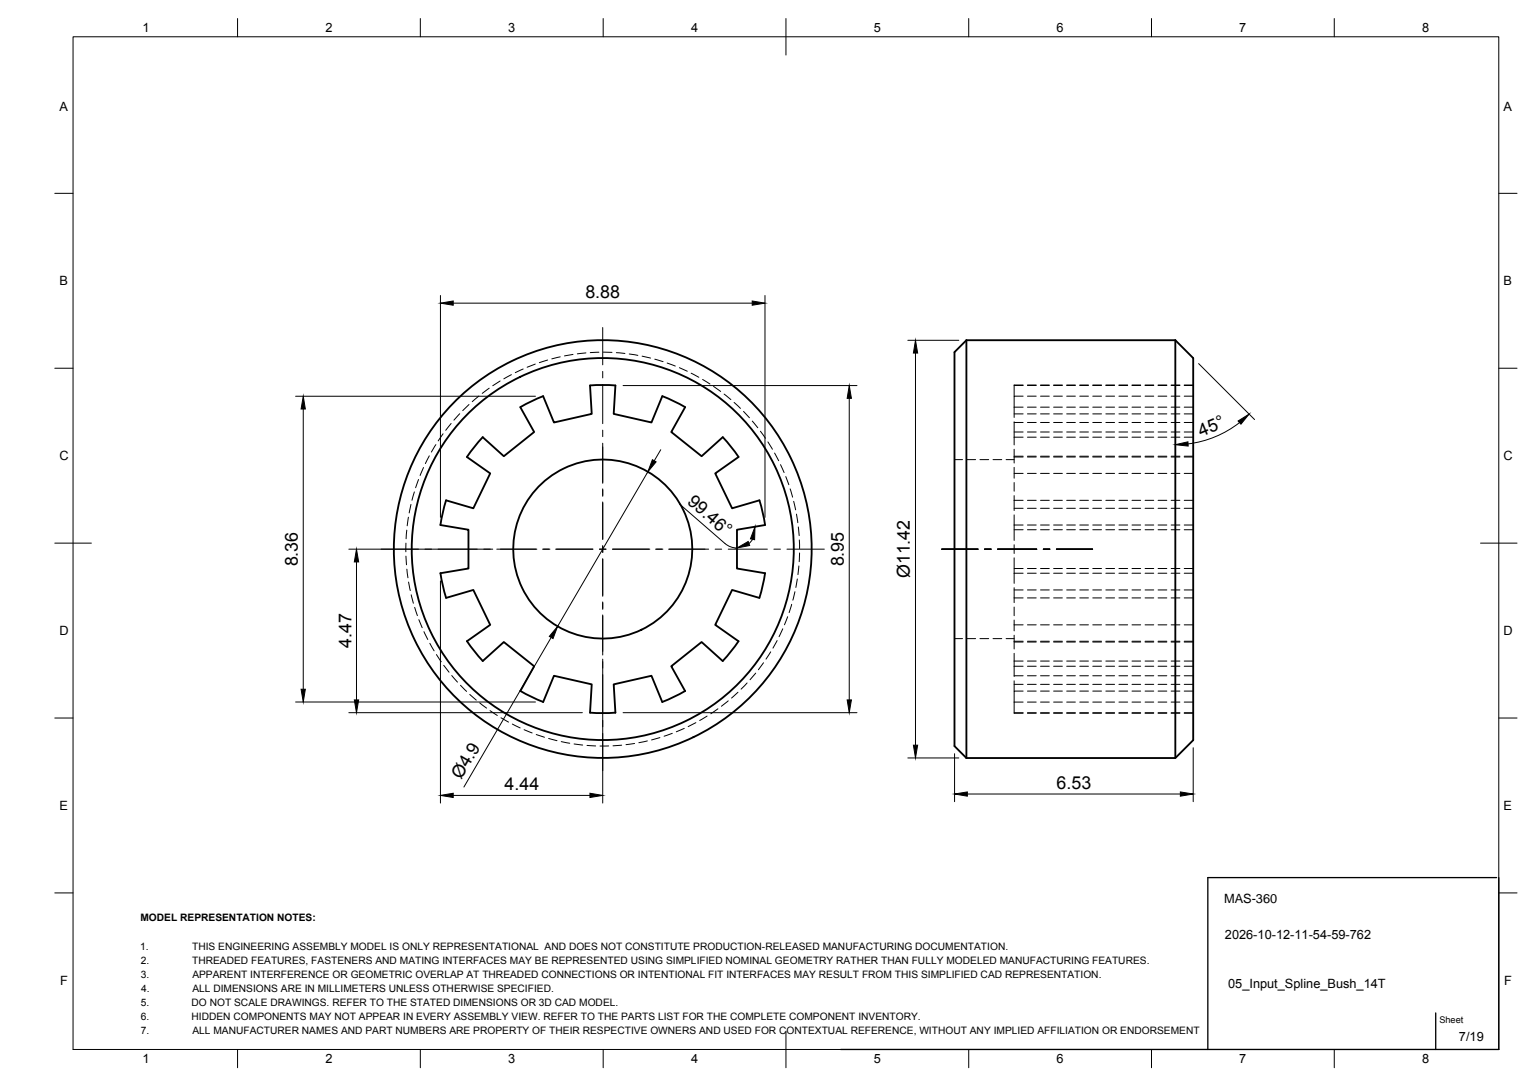
ISO-10303-21;
HEADER;
/* Generated by software containing ST-Developer
 * from STEP Tools, Inc. (www.steptools.com) 
 */

FILE_DESCRIPTION(
/* description */ (''),
/* implementation_level */ '2;1');

FILE_NAME(
/* name */ '05_Input_Spline_Bush_14T.step',
/* time_stamp */ '2026-11-04T18:53:29-08:00',
/* author */ (''),
/* organization */ (''),
/* preprocessor_version */ 'ST-DEVELOPER v20.2',
/* originating_system */ 'Autodesk Translation Framework v15.17.0.0',
/* authorisation */ '');

FILE_SCHEMA (('AUTOMOTIVE_DESIGN { 1 0 10303 214 3 1 1 }'));
ENDSEC;

DATA;
#10=MECHANICAL_DESIGN_GEOMETRIC_PRESENTATION_REPRESENTATION('',(#1331),#100031);
#230=CONICAL_SURFACE('',#21438,5.5488,0.785398163397448);
#231=CONICAL_SURFACE('',#21447,5.4672,0.785398163397448);
#748=CIRCLE('',#21439,5.712);
#749=CIRCLE('',#21440,5.3856);
#750=CIRCLE('',#21441,5.712);
#751=CIRCLE('',#21443,5.712);
#752=CIRCLE('',#21444,5.712);
#753=CIRCLE('',#21446,2.448);
#754=CIRCLE('',#21448,5.2224);
#755=CIRCLE('',#21450,4.488);
#756=CIRCLE('',#21451,4.488);
#757=CIRCLE('',#21452,4.488);
#758=CIRCLE('',#21453,4.488);
#759=CIRCLE('',#21454,4.488);
#760=CIRCLE('',#21455,4.488);
#761=CIRCLE('',#21456,4.488);
#762=CIRCLE('',#21457,4.488);
#763=CIRCLE('',#21458,4.488);
#764=CIRCLE('',#21459,4.488);
#765=CIRCLE('',#21460,4.488);
#766=CIRCLE('',#21461,4.488);
#767=CIRCLE('',#21462,4.488);
#768=CIRCLE('',#21463,4.488);
#769=CIRCLE('',#21468,4.488);
#770=CIRCLE('',#21473,4.488);
#771=CIRCLE('',#21478,4.488);
#772=CIRCLE('',#21483,4.488);
#773=CIRCLE('',#21488,4.488);
#774=CIRCLE('',#21493,4.488);
#775=CIRCLE('',#21498,4.488);
#776=CIRCLE('',#21503,4.488);
#777=CIRCLE('',#21508,4.488);
#778=CIRCLE('',#21513,4.488);
#779=CIRCLE('',#21518,4.488);
#780=CIRCLE('',#21523,4.488);
#781=CIRCLE('',#21528,4.488);
#782=CIRCLE('',#21533,4.488);
#783=CIRCLE('',#21534,2.448);
#1295=SHAPE_REPRESENTATION_RELATIONSHIP('SRR','None',#100105,#1313);
#1313=ADVANCED_BREP_SHAPE_REPRESENTATION('',(#1349),#100017);
#1331=STYLED_ITEM('',(#100200),#1349);
#1349=MANIFOLD_SOLID_BREP('Body1',#20121);
#1477=PLANE('',#21445);
#1478=PLANE('',#21449);
#1479=PLANE('',#21464);
#1480=PLANE('',#21465);
#1481=PLANE('',#21466);
#1482=PLANE('',#21469);
#1483=PLANE('',#21470);
#1484=PLANE('',#21471);
#1485=PLANE('',#21474);
#1486=PLANE('',#21475);
#1487=PLANE('',#21476);
#1488=PLANE('',#21479);
#1489=PLANE('',#21480);
#1490=PLANE('',#21481);
#1491=PLANE('',#21484);
#1492=PLANE('',#21485);
#1493=PLANE('',#21486);
#1494=PLANE('',#21489);
#1495=PLANE('',#21490);
#1496=PLANE('',#21491);
#1497=PLANE('',#21494);
#1498=PLANE('',#21495);
#1499=PLANE('',#21496);
#1500=PLANE('',#21499);
#1501=PLANE('',#21500);
#1502=PLANE('',#21501);
#1503=PLANE('',#21504);
#1504=PLANE('',#21505);
#1505=PLANE('',#21506);
#1506=PLANE('',#21509);
#1507=PLANE('',#21510);
#1508=PLANE('',#21511);
#1509=PLANE('',#21514);
#1510=PLANE('',#21515);
#1511=PLANE('',#21516);
#1512=PLANE('',#21519);
#1513=PLANE('',#21520);
#1514=PLANE('',#21521);
#1515=PLANE('',#21524);
#1516=PLANE('',#21525);
#1517=PLANE('',#21526);
#1518=PLANE('',#21529);
#1519=PLANE('',#21530);
#1520=PLANE('',#21531);
#1521=PLANE('',#21532);
#1754=FACE_BOUND('',#6840,.T.);
#1755=FACE_BOUND('',#6843,.T.);
#1756=FACE_BOUND('',#6900,.T.);
#2596=LINE('',#61632,#3883);
#2597=LINE('',#61640,#3884);
#2598=LINE('',#61646,#3885);
#2599=LINE('',#61653,#3886);
#2600=LINE('',#61655,#3887);
#2601=LINE('',#61657,#3888);
#2602=LINE('',#61661,#3889);
#2603=LINE('',#61663,#3890);
#2604=LINE('',#61665,#3891);
#2605=LINE('',#61669,#3892);
#2606=LINE('',#61671,#3893);
#2607=LINE('',#61673,#3894);
#2608=LINE('',#61677,#3895);
#2609=LINE('',#61679,#3896);
#2610=LINE('',#61681,#3897);
#2611=LINE('',#61685,#3898);
#2612=LINE('',#61687,#3899);
#2613=LINE('',#61689,#3900);
#2614=LINE('',#61693,#3901);
#2615=LINE('',#61695,#3902);
#2616=LINE('',#61697,#3903);
#2617=LINE('',#61701,#3904);
#2618=LINE('',#61703,#3905);
#2619=LINE('',#61705,#3906);
#2620=LINE('',#61709,#3907);
#2621=LINE('',#61711,#3908);
#2622=LINE('',#61713,#3909);
#2623=LINE('',#61717,#3910);
#2624=LINE('',#61719,#3911);
#2625=LINE('',#61721,#3912);
#2626=LINE('',#61725,#3913);
#2627=LINE('',#61727,#3914);
#2628=LINE('',#61729,#3915);
#2629=LINE('',#61733,#3916);
#2630=LINE('',#61735,#3917);
#2631=LINE('',#61737,#3918);
#2632=LINE('',#61741,#3919);
#2633=LINE('',#61743,#3920);
#2634=LINE('',#61745,#3921);
#2635=LINE('',#61749,#3922);
#2636=LINE('',#61751,#3923);
#2637=LINE('',#61753,#3924);
#2638=LINE('',#61757,#3925);
#2639=LINE('',#61759,#3926);
#2640=LINE('',#61760,#3927);
#2641=LINE('',#61763,#3928);
#2642=LINE('',#61765,#3929);
#2643=LINE('',#61766,#3930);
#2644=LINE('',#61769,#3931);
#2645=LINE('',#61771,#3932);
#2646=LINE('',#61772,#3933);
#2647=LINE('',#61774,#3934);
#2648=LINE('',#61778,#3935);
#2649=LINE('',#61781,#3936);
#2650=LINE('',#61782,#3937);
#2651=LINE('',#61785,#3938);
#2652=LINE('',#61787,#3939);
#2653=LINE('',#61788,#3940);
#2654=LINE('',#61790,#3941);
#2655=LINE('',#61794,#3942);
#2656=LINE('',#61797,#3943);
#2657=LINE('',#61798,#3944);
#2658=LINE('',#61801,#3945);
#2659=LINE('',#61803,#3946);
#2660=LINE('',#61804,#3947);
#2661=LINE('',#61806,#3948);
#2662=LINE('',#61810,#3949);
#2663=LINE('',#61813,#3950);
#2664=LINE('',#61814,#3951);
#2665=LINE('',#61817,#3952);
#2666=LINE('',#61819,#3953);
#2667=LINE('',#61820,#3954);
#2668=LINE('',#61822,#3955);
#2669=LINE('',#61826,#3956);
#2670=LINE('',#61829,#3957);
#2671=LINE('',#61830,#3958);
#2672=LINE('',#61833,#3959);
#2673=LINE('',#61835,#3960);
#2674=LINE('',#61836,#3961);
#2675=LINE('',#61838,#3962);
#2676=LINE('',#61842,#3963);
#2677=LINE('',#61845,#3964);
#2678=LINE('',#61846,#3965);
#2679=LINE('',#61849,#3966);
#2680=LINE('',#61851,#3967);
#2681=LINE('',#61852,#3968);
#2682=LINE('',#61854,#3969);
#2683=LINE('',#61858,#3970);
#2684=LINE('',#61861,#3971);
#2685=LINE('',#61862,#3972);
#2686=LINE('',#61865,#3973);
#2687=LINE('',#61867,#3974);
#2688=LINE('',#61868,#3975);
#2689=LINE('',#61870,#3976);
#2690=LINE('',#61874,#3977);
#2691=LINE('',#61877,#3978);
#2692=LINE('',#61878,#3979);
#2693=LINE('',#61881,#3980);
#2694=LINE('',#61883,#3981);
#2695=LINE('',#61884,#3982);
#2696=LINE('',#61886,#3983);
#2697=LINE('',#61890,#3984);
#2698=LINE('',#61893,#3985);
#2699=LINE('',#61894,#3986);
#2700=LINE('',#61897,#3987);
#2701=LINE('',#61899,#3988);
#2702=LINE('',#61900,#3989);
#2703=LINE('',#61902,#3990);
#2704=LINE('',#61906,#3991);
#2705=LINE('',#61909,#3992);
#2706=LINE('',#61910,#3993);
#2707=LINE('',#61913,#3994);
#2708=LINE('',#61915,#3995);
#2709=LINE('',#61916,#3996);
#2710=LINE('',#61918,#3997);
#2711=LINE('',#61922,#3998);
#2712=LINE('',#61925,#3999);
#2713=LINE('',#61926,#4000);
#2714=LINE('',#61929,#4001);
#2715=LINE('',#61931,#4002);
#2716=LINE('',#61932,#4003);
#2717=LINE('',#61934,#4004);
#2718=LINE('',#61938,#4005);
#2719=LINE('',#61941,#4006);
#2720=LINE('',#61942,#4007);
#2721=LINE('',#61945,#4008);
#2722=LINE('',#61947,#4009);
#2723=LINE('',#61948,#4010);
#2724=LINE('',#61950,#4011);
#2725=LINE('',#61954,#4012);
#2726=LINE('',#61957,#4013);
#2727=LINE('',#61958,#4014);
#2728=LINE('',#61961,#4015);
#2729=LINE('',#61963,#4016);
#2730=LINE('',#61964,#4017);
#2731=LINE('',#61966,#4018);
#2732=LINE('',#61970,#4019);
#2733=LINE('',#61973,#4020);
#2734=LINE('',#61975,#4021);
#2735=LINE('',#61976,#4022);
#2736=LINE('',#61979,#4023);
#2737=LINE('',#61980,#4024);
#2738=LINE('',#61982,#4025);
#2739=LINE('',#61989,#4026);
#3883=VECTOR('',#25353,5.5488);
#3884=VECTOR('',#25364,5.712);
#3885=VECTOR('',#25371,5.4672);
#3886=VECTOR('',#25378,10.);
#3887=VECTOR('',#25379,10.);
#3888=VECTOR('',#25380,10.);
#3889=VECTOR('',#25383,10.);
#3890=VECTOR('',#25384,10.);
#3891=VECTOR('',#25385,10.);
#3892=VECTOR('',#25388,10.);
#3893=VECTOR('',#25389,10.);
#3894=VECTOR('',#25390,10.);
#3895=VECTOR('',#25393,10.);
#3896=VECTOR('',#25394,10.);
#3897=VECTOR('',#25395,10.);
#3898=VECTOR('',#25398,10.);
#3899=VECTOR('',#25399,10.);
#3900=VECTOR('',#25400,10.);
#3901=VECTOR('',#25403,10.);
#3902=VECTOR('',#25404,10.);
#3903=VECTOR('',#25405,10.);
#3904=VECTOR('',#25408,10.);
#3905=VECTOR('',#25409,10.);
#3906=VECTOR('',#25410,10.);
#3907=VECTOR('',#25413,10.);
#3908=VECTOR('',#25414,10.);
#3909=VECTOR('',#25415,10.);
#3910=VECTOR('',#25418,10.);
#3911=VECTOR('',#25419,10.);
#3912=VECTOR('',#25420,10.);
#3913=VECTOR('',#25423,10.);
#3914=VECTOR('',#25424,10.);
#3915=VECTOR('',#25425,10.);
#3916=VECTOR('',#25428,10.);
#3917=VECTOR('',#25429,10.);
#3918=VECTOR('',#25430,10.);
#3919=VECTOR('',#25433,10.);
#3920=VECTOR('',#25434,10.);
#3921=VECTOR('',#25435,10.);
#3922=VECTOR('',#25438,10.);
#3923=VECTOR('',#25439,10.);
#3924=VECTOR('',#25440,10.);
#3925=VECTOR('',#25443,10.);
#3926=VECTOR('',#25444,10.);
#3927=VECTOR('',#25445,10.);
#3928=VECTOR('',#25448,10.);
#3929=VECTOR('',#25449,10.);
#3930=VECTOR('',#25450,10.);
#3931=VECTOR('',#25453,10.);
#3932=VECTOR('',#25454,10.);
#3933=VECTOR('',#25455,10.);
#3934=VECTOR('',#25458,10.);
#3935=VECTOR('',#25463,10.);
#3936=VECTOR('',#25466,10.);
#3937=VECTOR('',#25467,10.);
#3938=VECTOR('',#25470,10.);
#3939=VECTOR('',#25471,10.);
#3940=VECTOR('',#25472,10.);
#3941=VECTOR('',#25475,10.);
#3942=VECTOR('',#25480,10.);
#3943=VECTOR('',#25483,10.);
#3944=VECTOR('',#25484,10.);
#3945=VECTOR('',#25487,10.);
#3946=VECTOR('',#25488,10.);
#3947=VECTOR('',#25489,10.);
#3948=VECTOR('',#25492,10.);
#3949=VECTOR('',#25497,10.);
#3950=VECTOR('',#25500,10.);
#3951=VECTOR('',#25501,10.);
#3952=VECTOR('',#25504,10.);
#3953=VECTOR('',#25505,10.);
#3954=VECTOR('',#25506,10.);
#3955=VECTOR('',#25509,10.);
#3956=VECTOR('',#25514,10.);
#3957=VECTOR('',#25517,10.);
#3958=VECTOR('',#25518,10.);
#3959=VECTOR('',#25521,10.);
#3960=VECTOR('',#25522,10.);
#3961=VECTOR('',#25523,10.);
#3962=VECTOR('',#25526,10.);
#3963=VECTOR('',#25531,10.);
#3964=VECTOR('',#25534,10.);
#3965=VECTOR('',#25535,10.);
#3966=VECTOR('',#25538,10.);
#3967=VECTOR('',#25539,10.);
#3968=VECTOR('',#25540,10.);
#3969=VECTOR('',#25543,10.);
#3970=VECTOR('',#25548,10.);
#3971=VECTOR('',#25551,10.);
#3972=VECTOR('',#25552,10.);
#3973=VECTOR('',#25555,10.);
#3974=VECTOR('',#25556,10.);
#3975=VECTOR('',#25557,10.);
#3976=VECTOR('',#25560,10.);
#3977=VECTOR('',#25565,10.);
#3978=VECTOR('',#25568,10.);
#3979=VECTOR('',#25569,10.);
#3980=VECTOR('',#25572,10.);
#3981=VECTOR('',#25573,10.);
#3982=VECTOR('',#25574,10.);
#3983=VECTOR('',#25577,10.);
#3984=VECTOR('',#25582,10.);
#3985=VECTOR('',#25585,10.);
#3986=VECTOR('',#25586,10.);
#3987=VECTOR('',#25589,10.);
#3988=VECTOR('',#25590,10.);
#3989=VECTOR('',#25591,10.);
#3990=VECTOR('',#25594,10.);
#3991=VECTOR('',#25599,10.);
#3992=VECTOR('',#25602,10.);
#3993=VECTOR('',#25603,10.);
#3994=VECTOR('',#25606,10.);
#3995=VECTOR('',#25607,10.);
#3996=VECTOR('',#25608,10.);
#3997=VECTOR('',#25611,10.);
#3998=VECTOR('',#25616,10.);
#3999=VECTOR('',#25619,10.);
#4000=VECTOR('',#25620,10.);
#4001=VECTOR('',#25623,10.);
#4002=VECTOR('',#25624,10.);
#4003=VECTOR('',#25625,10.);
#4004=VECTOR('',#25628,10.);
#4005=VECTOR('',#25633,10.);
#4006=VECTOR('',#25636,10.);
#4007=VECTOR('',#25637,10.);
#4008=VECTOR('',#25640,10.);
#4009=VECTOR('',#25641,10.);
#4010=VECTOR('',#25642,10.);
#4011=VECTOR('',#25645,10.);
#4012=VECTOR('',#25650,10.);
#4013=VECTOR('',#25653,10.);
#4014=VECTOR('',#25654,10.);
#4015=VECTOR('',#25657,10.);
#4016=VECTOR('',#25658,10.);
#4017=VECTOR('',#25659,10.);
#4018=VECTOR('',#25662,10.);
#4019=VECTOR('',#25667,10.);
#4020=VECTOR('',#25670,10.);
#4021=VECTOR('',#25671,10.);
#4022=VECTOR('',#25672,10.);
#4023=VECTOR('',#25675,10.);
#4024=VECTOR('',#25676,10.);
#4025=VECTOR('',#25679,10.);
#4026=VECTOR('',#25690,2.448);
#4801=CYLINDRICAL_SURFACE('',#21442,5.712);
#4802=CYLINDRICAL_SURFACE('',#21467,4.488);
#4803=CYLINDRICAL_SURFACE('',#21472,4.488);
#4804=CYLINDRICAL_SURFACE('',#21477,4.488);
#4805=CYLINDRICAL_SURFACE('',#21482,4.488);
#4806=CYLINDRICAL_SURFACE('',#21487,4.488);
#4807=CYLINDRICAL_SURFACE('',#21492,4.488);
#4808=CYLINDRICAL_SURFACE('',#21497,4.488);
#4809=CYLINDRICAL_SURFACE('',#21502,4.488);
#4810=CYLINDRICAL_SURFACE('',#21507,4.488);
#4811=CYLINDRICAL_SURFACE('',#21512,4.488);
#4812=CYLINDRICAL_SURFACE('',#21517,4.488);
#4813=CYLINDRICAL_SURFACE('',#21522,4.488);
#4814=CYLINDRICAL_SURFACE('',#21527,4.488);
#4815=CYLINDRICAL_SURFACE('',#21535,4.488);
#4816=CYLINDRICAL_SURFACE('',#21536,2.448);
#5620=FACE_OUTER_BOUND('',#6837,.T.);
#5621=FACE_OUTER_BOUND('',#6838,.T.);
#5622=FACE_OUTER_BOUND('',#6839,.T.);
#5623=FACE_OUTER_BOUND('',#6841,.T.);
#5624=FACE_OUTER_BOUND('',#6842,.T.);
#5625=FACE_OUTER_BOUND('',#6844,.T.);
#5626=FACE_OUTER_BOUND('',#6845,.T.);
#5627=FACE_OUTER_BOUND('',#6846,.T.);
#5628=FACE_OUTER_BOUND('',#6847,.T.);
#5629=FACE_OUTER_BOUND('',#6848,.T.);
#5630=FACE_OUTER_BOUND('',#6849,.T.);
#5631=FACE_OUTER_BOUND('',#6850,.T.);
#5632=FACE_OUTER_BOUND('',#6851,.T.);
#5633=FACE_OUTER_BOUND('',#6852,.T.);
#5634=FACE_OUTER_BOUND('',#6853,.T.);
#5635=FACE_OUTER_BOUND('',#6854,.T.);
#5636=FACE_OUTER_BOUND('',#6855,.T.);
#5637=FACE_OUTER_BOUND('',#6856,.T.);
#5638=FACE_OUTER_BOUND('',#6857,.T.);
#5639=FACE_OUTER_BOUND('',#6858,.T.);
#5640=FACE_OUTER_BOUND('',#6859,.T.);
#5641=FACE_OUTER_BOUND('',#6860,.T.);
#5642=FACE_OUTER_BOUND('',#6861,.T.);
#5643=FACE_OUTER_BOUND('',#6862,.T.);
#5644=FACE_OUTER_BOUND('',#6863,.T.);
#5645=FACE_OUTER_BOUND('',#6864,.T.);
#5646=FACE_OUTER_BOUND('',#6865,.T.);
#5647=FACE_OUTER_BOUND('',#6866,.T.);
#5648=FACE_OUTER_BOUND('',#6867,.T.);
#5649=FACE_OUTER_BOUND('',#6868,.T.);
#5650=FACE_OUTER_BOUND('',#6869,.T.);
#5651=FACE_OUTER_BOUND('',#6870,.T.);
#5652=FACE_OUTER_BOUND('',#6871,.T.);
#5653=FACE_OUTER_BOUND('',#6872,.T.);
#5654=FACE_OUTER_BOUND('',#6873,.T.);
#5655=FACE_OUTER_BOUND('',#6874,.T.);
#5656=FACE_OUTER_BOUND('',#6875,.T.);
#5657=FACE_OUTER_BOUND('',#6876,.T.);
#5658=FACE_OUTER_BOUND('',#6877,.T.);
#5659=FACE_OUTER_BOUND('',#6878,.T.);
#5660=FACE_OUTER_BOUND('',#6879,.T.);
#5661=FACE_OUTER_BOUND('',#6880,.T.);
#5662=FACE_OUTER_BOUND('',#6881,.T.);
#5663=FACE_OUTER_BOUND('',#6882,.T.);
#5664=FACE_OUTER_BOUND('',#6883,.T.);
#5665=FACE_OUTER_BOUND('',#6884,.T.);
#5666=FACE_OUTER_BOUND('',#6885,.T.);
#5667=FACE_OUTER_BOUND('',#6886,.T.);
#5668=FACE_OUTER_BOUND('',#6887,.T.);
#5669=FACE_OUTER_BOUND('',#6888,.T.);
#5670=FACE_OUTER_BOUND('',#6889,.T.);
#5671=FACE_OUTER_BOUND('',#6890,.T.);
#5672=FACE_OUTER_BOUND('',#6891,.T.);
#5673=FACE_OUTER_BOUND('',#6892,.T.);
#5674=FACE_OUTER_BOUND('',#6893,.T.);
#5675=FACE_OUTER_BOUND('',#6894,.T.);
#5676=FACE_OUTER_BOUND('',#6895,.T.);
#5677=FACE_OUTER_BOUND('',#6896,.T.);
#5678=FACE_OUTER_BOUND('',#6897,.T.);
#5679=FACE_OUTER_BOUND('',#6898,.T.);
#5680=FACE_OUTER_BOUND('',#6899,.T.);
#5681=FACE_OUTER_BOUND('',#6901,.T.);
#5682=FACE_OUTER_BOUND('',#6902,.T.);
#6837=EDGE_LOOP('',(#15791,#15792,#15793,#15794,#15795));
#6838=EDGE_LOOP('',(#15796,#15797,#15798,#15799,#15800,#15801));
#6839=EDGE_LOOP('',(#15802));
#6840=EDGE_LOOP('',(#15803));
#6841=EDGE_LOOP('',(#15804,#15805,#15806,#15807,#15808));
#6842=EDGE_LOOP('',(#15809));
#6843=EDGE_LOOP('',(#15810,#15811,#15812,#15813,#15814,#15815,#15816,#15817,
#15818,#15819,#15820,#15821,#15822,#15823,#15824,#15825,#15826,#15827,#15828,
#15829,#15830,#15831,#15832,#15833,#15834,#15835,#15836,#15837,#15838,#15839,
#15840,#15841,#15842,#15843,#15844,#15845,#15846,#15847,#15848,#15849,#15850,
#15851,#15852,#15853,#15854,#15855,#15856,#15857,#15858,#15859,#15860,#15861,
#15862,#15863,#15864,#15865));
#6844=EDGE_LOOP('',(#15866,#15867,#15868,#15869));
#6845=EDGE_LOOP('',(#15870,#15871,#15872,#15873));
#6846=EDGE_LOOP('',(#15874,#15875,#15876,#15877));
#6847=EDGE_LOOP('',(#15878,#15879,#15880,#15881));
#6848=EDGE_LOOP('',(#15882,#15883,#15884,#15885));
#6849=EDGE_LOOP('',(#15886,#15887,#15888,#15889));
#6850=EDGE_LOOP('',(#15890,#15891,#15892,#15893));
#6851=EDGE_LOOP('',(#15894,#15895,#15896,#15897));
#6852=EDGE_LOOP('',(#15898,#15899,#15900,#15901));
#6853=EDGE_LOOP('',(#15902,#15903,#15904,#15905));
#6854=EDGE_LOOP('',(#15906,#15907,#15908,#15909));
#6855=EDGE_LOOP('',(#15910,#15911,#15912,#15913));
#6856=EDGE_LOOP('',(#15914,#15915,#15916,#15917));
#6857=EDGE_LOOP('',(#15918,#15919,#15920,#15921));
#6858=EDGE_LOOP('',(#15922,#15923,#15924,#15925));
#6859=EDGE_LOOP('',(#15926,#15927,#15928,#15929));
#6860=EDGE_LOOP('',(#15930,#15931,#15932,#15933));
#6861=EDGE_LOOP('',(#15934,#15935,#15936,#15937));
#6862=EDGE_LOOP('',(#15938,#15939,#15940,#15941));
#6863=EDGE_LOOP('',(#15942,#15943,#15944,#15945));
#6864=EDGE_LOOP('',(#15946,#15947,#15948,#15949));
#6865=EDGE_LOOP('',(#15950,#15951,#15952,#15953));
#6866=EDGE_LOOP('',(#15954,#15955,#15956,#15957));
#6867=EDGE_LOOP('',(#15958,#15959,#15960,#15961));
#6868=EDGE_LOOP('',(#15962,#15963,#15964,#15965));
#6869=EDGE_LOOP('',(#15966,#15967,#15968,#15969));
#6870=EDGE_LOOP('',(#15970,#15971,#15972,#15973));
#6871=EDGE_LOOP('',(#15974,#15975,#15976,#15977));
#6872=EDGE_LOOP('',(#15978,#15979,#15980,#15981));
#6873=EDGE_LOOP('',(#15982,#15983,#15984,#15985));
#6874=EDGE_LOOP('',(#15986,#15987,#15988,#15989));
#6875=EDGE_LOOP('',(#15990,#15991,#15992,#15993));
#6876=EDGE_LOOP('',(#15994,#15995,#15996,#15997));
#6877=EDGE_LOOP('',(#15998,#15999,#16000,#16001));
#6878=EDGE_LOOP('',(#16002,#16003,#16004,#16005));
#6879=EDGE_LOOP('',(#16006,#16007,#16008,#16009));
#6880=EDGE_LOOP('',(#16010,#16011,#16012,#16013));
#6881=EDGE_LOOP('',(#16014,#16015,#16016,#16017));
#6882=EDGE_LOOP('',(#16018,#16019,#16020,#16021));
#6883=EDGE_LOOP('',(#16022,#16023,#16024,#16025));
#6884=EDGE_LOOP('',(#16026,#16027,#16028,#16029));
#6885=EDGE_LOOP('',(#16030,#16031,#16032,#16033));
#6886=EDGE_LOOP('',(#16034,#16035,#16036,#16037));
#6887=EDGE_LOOP('',(#16038,#16039,#16040,#16041));
#6888=EDGE_LOOP('',(#16042,#16043,#16044,#16045));
#6889=EDGE_LOOP('',(#16046,#16047,#16048,#16049));
#6890=EDGE_LOOP('',(#16050,#16051,#16052,#16053));
#6891=EDGE_LOOP('',(#16054,#16055,#16056,#16057));
#6892=EDGE_LOOP('',(#16058,#16059,#16060,#16061));
#6893=EDGE_LOOP('',(#16062,#16063,#16064,#16065));
#6894=EDGE_LOOP('',(#16066,#16067,#16068,#16069));
#6895=EDGE_LOOP('',(#16070,#16071,#16072,#16073));
#6896=EDGE_LOOP('',(#16074,#16075,#16076,#16077));
#6897=EDGE_LOOP('',(#16078,#16079,#16080,#16081));
#6898=EDGE_LOOP('',(#16082,#16083,#16084,#16085));
#6899=EDGE_LOOP('',(#16086,#16087,#16088,#16089,#16090,#16091,#16092,#16093,
#16094,#16095,#16096,#16097,#16098,#16099,#16100,#16101,#16102,#16103,#16104,
#16105,#16106,#16107,#16108,#16109,#16110,#16111,#16112,#16113,#16114,#16115,
#16116,#16117,#16118,#16119,#16120,#16121,#16122,#16123,#16124,#16125,#16126,
#16127,#16128,#16129,#16130,#16131,#16132,#16133,#16134,#16135,#16136,#16137,
#16138,#16139,#16140,#16141));
#6900=EDGE_LOOP('',(#16142));
#6901=EDGE_LOOP('',(#16143,#16144,#16145,#16146));
#6902=EDGE_LOOP('',(#16147,#16148,#16149,#16150));
#8915=VERTEX_POINT('',#61628);
#8916=VERTEX_POINT('',#61629);
#8917=VERTEX_POINT('',#61631);
#8918=VERTEX_POINT('',#61636);
#8919=VERTEX_POINT('',#61637);
#8920=VERTEX_POINT('',#61642);
#8921=VERTEX_POINT('',#61645);
#8922=VERTEX_POINT('',#61649);
#8923=VERTEX_POINT('',#61650);
#8924=VERTEX_POINT('',#61652);
#8925=VERTEX_POINT('',#61654);
#8926=VERTEX_POINT('',#61656);
#8927=VERTEX_POINT('',#61658);
#8928=VERTEX_POINT('',#61660);
#8929=VERTEX_POINT('',#61662);
#8930=VERTEX_POINT('',#61664);
#8931=VERTEX_POINT('',#61666);
#8932=VERTEX_POINT('',#61668);
#8933=VERTEX_POINT('',#61670);
#8934=VERTEX_POINT('',#61672);
#8935=VERTEX_POINT('',#61674);
#8936=VERTEX_POINT('',#61676);
#8937=VERTEX_POINT('',#61678);
#8938=VERTEX_POINT('',#61680);
#8939=VERTEX_POINT('',#61682);
#8940=VERTEX_POINT('',#61684);
#8941=VERTEX_POINT('',#61686);
#8942=VERTEX_POINT('',#61688);
#8943=VERTEX_POINT('',#61690);
#8944=VERTEX_POINT('',#61692);
#8945=VERTEX_POINT('',#61694);
#8946=VERTEX_POINT('',#61696);
#8947=VERTEX_POINT('',#61698);
#8948=VERTEX_POINT('',#61700);
#8949=VERTEX_POINT('',#61702);
#8950=VERTEX_POINT('',#61704);
#8951=VERTEX_POINT('',#61706);
#8952=VERTEX_POINT('',#61708);
#8953=VERTEX_POINT('',#61710);
#8954=VERTEX_POINT('',#61712);
#8955=VERTEX_POINT('',#61714);
#8956=VERTEX_POINT('',#61716);
#8957=VERTEX_POINT('',#61718);
#8958=VERTEX_POINT('',#61720);
#8959=VERTEX_POINT('',#61722);
#8960=VERTEX_POINT('',#61724);
#8961=VERTEX_POINT('',#61726);
#8962=VERTEX_POINT('',#61728);
#8963=VERTEX_POINT('',#61730);
#8964=VERTEX_POINT('',#61732);
#8965=VERTEX_POINT('',#61734);
#8966=VERTEX_POINT('',#61736);
#8967=VERTEX_POINT('',#61738);
#8968=VERTEX_POINT('',#61740);
#8969=VERTEX_POINT('',#61742);
#8970=VERTEX_POINT('',#61744);
#8971=VERTEX_POINT('',#61746);
#8972=VERTEX_POINT('',#61748);
#8973=VERTEX_POINT('',#61750);
#8974=VERTEX_POINT('',#61752);
#8975=VERTEX_POINT('',#61754);
#8976=VERTEX_POINT('',#61756);
#8977=VERTEX_POINT('',#61758);
#8978=VERTEX_POINT('',#61762);
#8979=VERTEX_POINT('',#61764);
#8980=VERTEX_POINT('',#61768);
#8981=VERTEX_POINT('',#61770);
#8982=VERTEX_POINT('',#61776);
#8983=VERTEX_POINT('',#61780);
#8984=VERTEX_POINT('',#61784);
#8985=VERTEX_POINT('',#61786);
#8986=VERTEX_POINT('',#61792);
#8987=VERTEX_POINT('',#61796);
#8988=VERTEX_POINT('',#61800);
#8989=VERTEX_POINT('',#61802);
#8990=VERTEX_POINT('',#61808);
#8991=VERTEX_POINT('',#61812);
#8992=VERTEX_POINT('',#61816);
#8993=VERTEX_POINT('',#61818);
#8994=VERTEX_POINT('',#61824);
#8995=VERTEX_POINT('',#61828);
#8996=VERTEX_POINT('',#61832);
#8997=VERTEX_POINT('',#61834);
#8998=VERTEX_POINT('',#61840);
#8999=VERTEX_POINT('',#61844);
#9000=VERTEX_POINT('',#61848);
#9001=VERTEX_POINT('',#61850);
#9002=VERTEX_POINT('',#61856);
#9003=VERTEX_POINT('',#61860);
#9004=VERTEX_POINT('',#61864);
#9005=VERTEX_POINT('',#61866);
#9006=VERTEX_POINT('',#61872);
#9007=VERTEX_POINT('',#61876);
#9008=VERTEX_POINT('',#61880);
#9009=VERTEX_POINT('',#61882);
#9010=VERTEX_POINT('',#61888);
#9011=VERTEX_POINT('',#61892);
#9012=VERTEX_POINT('',#61896);
#9013=VERTEX_POINT('',#61898);
#9014=VERTEX_POINT('',#61904);
#9015=VERTEX_POINT('',#61908);
#9016=VERTEX_POINT('',#61912);
#9017=VERTEX_POINT('',#61914);
#9018=VERTEX_POINT('',#61920);
#9019=VERTEX_POINT('',#61924);
#9020=VERTEX_POINT('',#61928);
#9021=VERTEX_POINT('',#61930);
#9022=VERTEX_POINT('',#61936);
#9023=VERTEX_POINT('',#61940);
#9024=VERTEX_POINT('',#61944);
#9025=VERTEX_POINT('',#61946);
#9026=VERTEX_POINT('',#61952);
#9027=VERTEX_POINT('',#61956);
#9028=VERTEX_POINT('',#61960);
#9029=VERTEX_POINT('',#61962);
#9030=VERTEX_POINT('',#61968);
#9031=VERTEX_POINT('',#61972);
#9032=VERTEX_POINT('',#61974);
#9033=VERTEX_POINT('',#61978);
#9034=VERTEX_POINT('',#61985);
#11370=EDGE_CURVE('',#8915,#8916,#748,.T.);
#11371=EDGE_CURVE('',#8916,#8917,#2596,.T.);
#11372=EDGE_CURVE('',#8917,#8917,#749,.T.);
#11373=EDGE_CURVE('',#8916,#8915,#750,.T.);
#11374=EDGE_CURVE('',#8918,#8919,#751,.T.);
#11375=EDGE_CURVE('',#8919,#8918,#752,.T.);
#11376=EDGE_CURVE('',#8919,#8915,#2597,.T.);
#11377=EDGE_CURVE('',#8920,#8920,#753,.T.);
#11378=EDGE_CURVE('',#8918,#8921,#2598,.T.);
#11379=EDGE_CURVE('',#8921,#8921,#754,.T.);
#11380=EDGE_CURVE('',#8922,#8923,#755,.T.);
#11381=EDGE_CURVE('',#8923,#8924,#2599,.T.);
#11382=EDGE_CURVE('',#8924,#8925,#2600,.T.);
#11383=EDGE_CURVE('',#8925,#8926,#2601,.T.);
#11384=EDGE_CURVE('',#8926,#8927,#756,.T.);
#11385=EDGE_CURVE('',#8927,#8928,#2602,.T.);
#11386=EDGE_CURVE('',#8928,#8929,#2603,.T.);
#11387=EDGE_CURVE('',#8929,#8930,#2604,.T.);
#11388=EDGE_CURVE('',#8930,#8931,#757,.T.);
#11389=EDGE_CURVE('',#8931,#8932,#2605,.T.);
#11390=EDGE_CURVE('',#8932,#8933,#2606,.T.);
#11391=EDGE_CURVE('',#8933,#8934,#2607,.T.);
#11392=EDGE_CURVE('',#8934,#8935,#758,.T.);
#11393=EDGE_CURVE('',#8935,#8936,#2608,.T.);
#11394=EDGE_CURVE('',#8936,#8937,#2609,.T.);
#11395=EDGE_CURVE('',#8937,#8938,#2610,.T.);
#11396=EDGE_CURVE('',#8938,#8939,#759,.T.);
#11397=EDGE_CURVE('',#8939,#8940,#2611,.T.);
#11398=EDGE_CURVE('',#8940,#8941,#2612,.T.);
#11399=EDGE_CURVE('',#8941,#8942,#2613,.T.);
#11400=EDGE_CURVE('',#8942,#8943,#760,.T.);
#11401=EDGE_CURVE('',#8943,#8944,#2614,.T.);
#11402=EDGE_CURVE('',#8944,#8945,#2615,.T.);
#11403=EDGE_CURVE('',#8945,#8946,#2616,.T.);
#11404=EDGE_CURVE('',#8946,#8947,#761,.T.);
#11405=EDGE_CURVE('',#8947,#8948,#2617,.T.);
#11406=EDGE_CURVE('',#8948,#8949,#2618,.T.);
#11407=EDGE_CURVE('',#8949,#8950,#2619,.T.);
#11408=EDGE_CURVE('',#8950,#8951,#762,.T.);
#11409=EDGE_CURVE('',#8951,#8952,#2620,.T.);
#11410=EDGE_CURVE('',#8952,#8953,#2621,.T.);
#11411=EDGE_CURVE('',#8953,#8954,#2622,.T.);
#11412=EDGE_CURVE('',#8954,#8955,#763,.T.);
#11413=EDGE_CURVE('',#8955,#8956,#2623,.T.);
#11414=EDGE_CURVE('',#8956,#8957,#2624,.T.);
#11415=EDGE_CURVE('',#8957,#8958,#2625,.T.);
#11416=EDGE_CURVE('',#8958,#8959,#764,.T.);
#11417=EDGE_CURVE('',#8959,#8960,#2626,.T.);
#11418=EDGE_CURVE('',#8960,#8961,#2627,.T.);
#11419=EDGE_CURVE('',#8961,#8962,#2628,.T.);
#11420=EDGE_CURVE('',#8962,#8963,#765,.T.);
#11421=EDGE_CURVE('',#8963,#8964,#2629,.T.);
#11422=EDGE_CURVE('',#8964,#8965,#2630,.T.);
#11423=EDGE_CURVE('',#8965,#8966,#2631,.T.);
#11424=EDGE_CURVE('',#8966,#8967,#766,.T.);
#11425=EDGE_CURVE('',#8967,#8968,#2632,.T.);
#11426=EDGE_CURVE('',#8968,#8969,#2633,.T.);
#11427=EDGE_CURVE('',#8969,#8970,#2634,.T.);
#11428=EDGE_CURVE('',#8970,#8971,#767,.T.);
#11429=EDGE_CURVE('',#8971,#8972,#2635,.T.);
#11430=EDGE_CURVE('',#8972,#8973,#2636,.T.);
#11431=EDGE_CURVE('',#8973,#8974,#2637,.T.);
#11432=EDGE_CURVE('',#8974,#8975,#768,.T.);
#11433=EDGE_CURVE('',#8975,#8976,#2638,.T.);
#11434=EDGE_CURVE('',#8976,#8977,#2639,.T.);
#11435=EDGE_CURVE('',#8977,#8922,#2640,.T.);
#11436=EDGE_CURVE('',#8978,#8975,#2641,.T.);
#11437=EDGE_CURVE('',#8979,#8978,#2642,.T.);
#11438=EDGE_CURVE('',#8979,#8976,#2643,.T.);
#11439=EDGE_CURVE('',#8922,#8980,#2644,.T.);
#11440=EDGE_CURVE('',#8981,#8977,#2645,.T.);
#11441=EDGE_CURVE('',#8980,#8981,#2646,.T.);
#11442=EDGE_CURVE('',#8981,#8979,#2647,.T.);
#11443=EDGE_CURVE('',#8982,#8980,#769,.T.);
#11444=EDGE_CURVE('',#8982,#8923,#2648,.T.);
#11445=EDGE_CURVE('',#8983,#8982,#2649,.T.);
#11446=EDGE_CURVE('',#8983,#8924,#2650,.T.);
#11447=EDGE_CURVE('',#8926,#8984,#2651,.T.);
#11448=EDGE_CURVE('',#8985,#8925,#2652,.T.);
#11449=EDGE_CURVE('',#8984,#8985,#2653,.T.);
#11450=EDGE_CURVE('',#8985,#8983,#2654,.T.);
#11451=EDGE_CURVE('',#8986,#8984,#770,.T.);
#11452=EDGE_CURVE('',#8986,#8927,#2655,.T.);
#11453=EDGE_CURVE('',#8987,#8986,#2656,.T.);
#11454=EDGE_CURVE('',#8987,#8928,#2657,.T.);
#11455=EDGE_CURVE('',#8930,#8988,#2658,.T.);
#11456=EDGE_CURVE('',#8989,#8929,#2659,.T.);
#11457=EDGE_CURVE('',#8988,#8989,#2660,.T.);
#11458=EDGE_CURVE('',#8989,#8987,#2661,.T.);
#11459=EDGE_CURVE('',#8990,#8988,#771,.T.);
#11460=EDGE_CURVE('',#8990,#8931,#2662,.T.);
#11461=EDGE_CURVE('',#8991,#8990,#2663,.T.);
#11462=EDGE_CURVE('',#8991,#8932,#2664,.T.);
#11463=EDGE_CURVE('',#8934,#8992,#2665,.T.);
#11464=EDGE_CURVE('',#8993,#8933,#2666,.T.);
#11465=EDGE_CURVE('',#8992,#8993,#2667,.T.);
#11466=EDGE_CURVE('',#8993,#8991,#2668,.T.);
#11467=EDGE_CURVE('',#8994,#8992,#772,.T.);
#11468=EDGE_CURVE('',#8994,#8935,#2669,.T.);
#11469=EDGE_CURVE('',#8995,#8994,#2670,.T.);
#11470=EDGE_CURVE('',#8995,#8936,#2671,.T.);
#11471=EDGE_CURVE('',#8938,#8996,#2672,.T.);
#11472=EDGE_CURVE('',#8997,#8937,#2673,.T.);
#11473=EDGE_CURVE('',#8996,#8997,#2674,.T.);
#11474=EDGE_CURVE('',#8997,#8995,#2675,.T.);
#11475=EDGE_CURVE('',#8998,#8996,#773,.T.);
#11476=EDGE_CURVE('',#8998,#8939,#2676,.T.);
#11477=EDGE_CURVE('',#8999,#8998,#2677,.T.);
#11478=EDGE_CURVE('',#8999,#8940,#2678,.T.);
#11479=EDGE_CURVE('',#8942,#9000,#2679,.T.);
#11480=EDGE_CURVE('',#9001,#8941,#2680,.T.);
#11481=EDGE_CURVE('',#9000,#9001,#2681,.T.);
#11482=EDGE_CURVE('',#9001,#8999,#2682,.T.);
#11483=EDGE_CURVE('',#9002,#9000,#774,.T.);
#11484=EDGE_CURVE('',#9002,#8943,#2683,.T.);
#11485=EDGE_CURVE('',#9003,#9002,#2684,.T.);
#11486=EDGE_CURVE('',#9003,#8944,#2685,.T.);
#11487=EDGE_CURVE('',#8946,#9004,#2686,.T.);
#11488=EDGE_CURVE('',#9005,#8945,#2687,.T.);
#11489=EDGE_CURVE('',#9004,#9005,#2688,.T.);
#11490=EDGE_CURVE('',#9005,#9003,#2689,.T.);
#11491=EDGE_CURVE('',#9006,#9004,#775,.T.);
#11492=EDGE_CURVE('',#9006,#8947,#2690,.T.);
#11493=EDGE_CURVE('',#9007,#9006,#2691,.T.);
#11494=EDGE_CURVE('',#9007,#8948,#2692,.T.);
#11495=EDGE_CURVE('',#8950,#9008,#2693,.T.);
#11496=EDGE_CURVE('',#9009,#8949,#2694,.T.);
#11497=EDGE_CURVE('',#9008,#9009,#2695,.T.);
#11498=EDGE_CURVE('',#9009,#9007,#2696,.T.);
#11499=EDGE_CURVE('',#9010,#9008,#776,.T.);
#11500=EDGE_CURVE('',#9010,#8951,#2697,.T.);
#11501=EDGE_CURVE('',#9011,#9010,#2698,.T.);
#11502=EDGE_CURVE('',#9011,#8952,#2699,.T.);
#11503=EDGE_CURVE('',#8954,#9012,#2700,.T.);
#11504=EDGE_CURVE('',#9013,#8953,#2701,.T.);
#11505=EDGE_CURVE('',#9012,#9013,#2702,.T.);
#11506=EDGE_CURVE('',#9013,#9011,#2703,.T.);
#11507=EDGE_CURVE('',#9014,#9012,#777,.T.);
#11508=EDGE_CURVE('',#9014,#8955,#2704,.T.);
#11509=EDGE_CURVE('',#9015,#9014,#2705,.T.);
#11510=EDGE_CURVE('',#9015,#8956,#2706,.T.);
#11511=EDGE_CURVE('',#8958,#9016,#2707,.T.);
#11512=EDGE_CURVE('',#9017,#8957,#2708,.T.);
#11513=EDGE_CURVE('',#9016,#9017,#2709,.T.);
#11514=EDGE_CURVE('',#9017,#9015,#2710,.T.);
#11515=EDGE_CURVE('',#9018,#9016,#778,.T.);
#11516=EDGE_CURVE('',#9018,#8959,#2711,.T.);
#11517=EDGE_CURVE('',#9019,#9018,#2712,.T.);
#11518=EDGE_CURVE('',#9019,#8960,#2713,.T.);
#11519=EDGE_CURVE('',#8962,#9020,#2714,.T.);
#11520=EDGE_CURVE('',#9021,#8961,#2715,.T.);
#11521=EDGE_CURVE('',#9020,#9021,#2716,.T.);
#11522=EDGE_CURVE('',#9021,#9019,#2717,.T.);
#11523=EDGE_CURVE('',#9022,#9020,#779,.T.);
#11524=EDGE_CURVE('',#9022,#8963,#2718,.T.);
#11525=EDGE_CURVE('',#9023,#9022,#2719,.T.);
#11526=EDGE_CURVE('',#9023,#8964,#2720,.T.);
#11527=EDGE_CURVE('',#8966,#9024,#2721,.T.);
#11528=EDGE_CURVE('',#9025,#8965,#2722,.T.);
#11529=EDGE_CURVE('',#9024,#9025,#2723,.T.);
#11530=EDGE_CURVE('',#9025,#9023,#2724,.T.);
#11531=EDGE_CURVE('',#9026,#9024,#780,.T.);
#11532=EDGE_CURVE('',#9026,#8967,#2725,.T.);
#11533=EDGE_CURVE('',#9027,#9026,#2726,.T.);
#11534=EDGE_CURVE('',#9027,#8968,#2727,.T.);
#11535=EDGE_CURVE('',#8970,#9028,#2728,.T.);
#11536=EDGE_CURVE('',#9029,#8969,#2729,.T.);
#11537=EDGE_CURVE('',#9028,#9029,#2730,.T.);
#11538=EDGE_CURVE('',#9029,#9027,#2731,.T.);
#11539=EDGE_CURVE('',#9030,#9028,#781,.T.);
#11540=EDGE_CURVE('',#9030,#8971,#2732,.T.);
#11541=EDGE_CURVE('',#8974,#9031,#2733,.T.);
#11542=EDGE_CURVE('',#9032,#8973,#2734,.T.);
#11543=EDGE_CURVE('',#9031,#9032,#2735,.T.);
#11544=EDGE_CURVE('',#9033,#9030,#2736,.T.);
#11545=EDGE_CURVE('',#9033,#8972,#2737,.T.);
#11546=EDGE_CURVE('',#9032,#9033,#2738,.T.);
#11547=EDGE_CURVE('',#8978,#9031,#782,.T.);
#11548=EDGE_CURVE('',#9034,#9034,#783,.T.);
#11549=EDGE_CURVE('',#8920,#9034,#2739,.T.);
#15791=ORIENTED_EDGE('',*,*,#11370,.T.);
#15792=ORIENTED_EDGE('',*,*,#11371,.T.);
#15793=ORIENTED_EDGE('',*,*,#11372,.T.);
#15794=ORIENTED_EDGE('',*,*,#11371,.F.);
#15795=ORIENTED_EDGE('',*,*,#11373,.T.);
#15796=ORIENTED_EDGE('',*,*,#11374,.F.);
#15797=ORIENTED_EDGE('',*,*,#11375,.F.);
#15798=ORIENTED_EDGE('',*,*,#11376,.T.);
#15799=ORIENTED_EDGE('',*,*,#11373,.F.);
#15800=ORIENTED_EDGE('',*,*,#11370,.F.);
#15801=ORIENTED_EDGE('',*,*,#11376,.F.);
#15802=ORIENTED_EDGE('',*,*,#11372,.F.);
#15803=ORIENTED_EDGE('',*,*,#11377,.T.);
#15804=ORIENTED_EDGE('',*,*,#11374,.T.);
#15805=ORIENTED_EDGE('',*,*,#11375,.T.);
#15806=ORIENTED_EDGE('',*,*,#11378,.T.);
#15807=ORIENTED_EDGE('',*,*,#11379,.T.);
#15808=ORIENTED_EDGE('',*,*,#11378,.F.);
#15809=ORIENTED_EDGE('',*,*,#11379,.F.);
#15810=ORIENTED_EDGE('',*,*,#11380,.T.);
#15811=ORIENTED_EDGE('',*,*,#11381,.T.);
#15812=ORIENTED_EDGE('',*,*,#11382,.T.);
#15813=ORIENTED_EDGE('',*,*,#11383,.T.);
#15814=ORIENTED_EDGE('',*,*,#11384,.T.);
#15815=ORIENTED_EDGE('',*,*,#11385,.T.);
#15816=ORIENTED_EDGE('',*,*,#11386,.T.);
#15817=ORIENTED_EDGE('',*,*,#11387,.T.);
#15818=ORIENTED_EDGE('',*,*,#11388,.T.);
#15819=ORIENTED_EDGE('',*,*,#11389,.T.);
#15820=ORIENTED_EDGE('',*,*,#11390,.T.);
#15821=ORIENTED_EDGE('',*,*,#11391,.T.);
#15822=ORIENTED_EDGE('',*,*,#11392,.T.);
#15823=ORIENTED_EDGE('',*,*,#11393,.T.);
#15824=ORIENTED_EDGE('',*,*,#11394,.T.);
#15825=ORIENTED_EDGE('',*,*,#11395,.T.);
#15826=ORIENTED_EDGE('',*,*,#11396,.T.);
#15827=ORIENTED_EDGE('',*,*,#11397,.T.);
#15828=ORIENTED_EDGE('',*,*,#11398,.T.);
#15829=ORIENTED_EDGE('',*,*,#11399,.T.);
#15830=ORIENTED_EDGE('',*,*,#11400,.T.);
#15831=ORIENTED_EDGE('',*,*,#11401,.T.);
#15832=ORIENTED_EDGE('',*,*,#11402,.T.);
#15833=ORIENTED_EDGE('',*,*,#11403,.T.);
#15834=ORIENTED_EDGE('',*,*,#11404,.T.);
#15835=ORIENTED_EDGE('',*,*,#11405,.T.);
#15836=ORIENTED_EDGE('',*,*,#11406,.T.);
#15837=ORIENTED_EDGE('',*,*,#11407,.T.);
#15838=ORIENTED_EDGE('',*,*,#11408,.T.);
#15839=ORIENTED_EDGE('',*,*,#11409,.T.);
#15840=ORIENTED_EDGE('',*,*,#11410,.T.);
#15841=ORIENTED_EDGE('',*,*,#11411,.T.);
#15842=ORIENTED_EDGE('',*,*,#11412,.T.);
#15843=ORIENTED_EDGE('',*,*,#11413,.T.);
#15844=ORIENTED_EDGE('',*,*,#11414,.T.);
#15845=ORIENTED_EDGE('',*,*,#11415,.T.);
#15846=ORIENTED_EDGE('',*,*,#11416,.T.);
#15847=ORIENTED_EDGE('',*,*,#11417,.T.);
#15848=ORIENTED_EDGE('',*,*,#11418,.T.);
#15849=ORIENTED_EDGE('',*,*,#11419,.T.);
#15850=ORIENTED_EDGE('',*,*,#11420,.T.);
#15851=ORIENTED_EDGE('',*,*,#11421,.T.);
#15852=ORIENTED_EDGE('',*,*,#11422,.T.);
#15853=ORIENTED_EDGE('',*,*,#11423,.T.);
#15854=ORIENTED_EDGE('',*,*,#11424,.T.);
#15855=ORIENTED_EDGE('',*,*,#11425,.T.);
#15856=ORIENTED_EDGE('',*,*,#11426,.T.);
#15857=ORIENTED_EDGE('',*,*,#11427,.T.);
#15858=ORIENTED_EDGE('',*,*,#11428,.T.);
#15859=ORIENTED_EDGE('',*,*,#11429,.T.);
#15860=ORIENTED_EDGE('',*,*,#11430,.T.);
#15861=ORIENTED_EDGE('',*,*,#11431,.T.);
#15862=ORIENTED_EDGE('',*,*,#11432,.T.);
#15863=ORIENTED_EDGE('',*,*,#11433,.T.);
#15864=ORIENTED_EDGE('',*,*,#11434,.T.);
#15865=ORIENTED_EDGE('',*,*,#11435,.T.);
#15866=ORIENTED_EDGE('',*,*,#11436,.F.);
#15867=ORIENTED_EDGE('',*,*,#11437,.F.);
#15868=ORIENTED_EDGE('',*,*,#11438,.T.);
#15869=ORIENTED_EDGE('',*,*,#11433,.F.);
#15870=ORIENTED_EDGE('',*,*,#11439,.F.);
#15871=ORIENTED_EDGE('',*,*,#11435,.F.);
#15872=ORIENTED_EDGE('',*,*,#11440,.F.);
#15873=ORIENTED_EDGE('',*,*,#11441,.F.);
#15874=ORIENTED_EDGE('',*,*,#11442,.F.);
#15875=ORIENTED_EDGE('',*,*,#11440,.T.);
#15876=ORIENTED_EDGE('',*,*,#11434,.F.);
#15877=ORIENTED_EDGE('',*,*,#11438,.F.);
#15878=ORIENTED_EDGE('',*,*,#11439,.T.);
#15879=ORIENTED_EDGE('',*,*,#11443,.F.);
#15880=ORIENTED_EDGE('',*,*,#11444,.T.);
#15881=ORIENTED_EDGE('',*,*,#11380,.F.);
#15882=ORIENTED_EDGE('',*,*,#11444,.F.);
#15883=ORIENTED_EDGE('',*,*,#11445,.F.);
#15884=ORIENTED_EDGE('',*,*,#11446,.T.);
#15885=ORIENTED_EDGE('',*,*,#11381,.F.);
#15886=ORIENTED_EDGE('',*,*,#11447,.F.);
#15887=ORIENTED_EDGE('',*,*,#11383,.F.);
#15888=ORIENTED_EDGE('',*,*,#11448,.F.);
#15889=ORIENTED_EDGE('',*,*,#11449,.F.);
#15890=ORIENTED_EDGE('',*,*,#11450,.F.);
#15891=ORIENTED_EDGE('',*,*,#11448,.T.);
#15892=ORIENTED_EDGE('',*,*,#11382,.F.);
#15893=ORIENTED_EDGE('',*,*,#11446,.F.);
#15894=ORIENTED_EDGE('',*,*,#11447,.T.);
#15895=ORIENTED_EDGE('',*,*,#11451,.F.);
#15896=ORIENTED_EDGE('',*,*,#11452,.T.);
#15897=ORIENTED_EDGE('',*,*,#11384,.F.);
#15898=ORIENTED_EDGE('',*,*,#11452,.F.);
#15899=ORIENTED_EDGE('',*,*,#11453,.F.);
#15900=ORIENTED_EDGE('',*,*,#11454,.T.);
#15901=ORIENTED_EDGE('',*,*,#11385,.F.);
#15902=ORIENTED_EDGE('',*,*,#11455,.F.);
#15903=ORIENTED_EDGE('',*,*,#11387,.F.);
#15904=ORIENTED_EDGE('',*,*,#11456,.F.);
#15905=ORIENTED_EDGE('',*,*,#11457,.F.);
#15906=ORIENTED_EDGE('',*,*,#11458,.F.);
#15907=ORIENTED_EDGE('',*,*,#11456,.T.);
#15908=ORIENTED_EDGE('',*,*,#11386,.F.);
#15909=ORIENTED_EDGE('',*,*,#11454,.F.);
#15910=ORIENTED_EDGE('',*,*,#11455,.T.);
#15911=ORIENTED_EDGE('',*,*,#11459,.F.);
#15912=ORIENTED_EDGE('',*,*,#11460,.T.);
#15913=ORIENTED_EDGE('',*,*,#11388,.F.);
#15914=ORIENTED_EDGE('',*,*,#11460,.F.);
#15915=ORIENTED_EDGE('',*,*,#11461,.F.);
#15916=ORIENTED_EDGE('',*,*,#11462,.T.);
#15917=ORIENTED_EDGE('',*,*,#11389,.F.);
#15918=ORIENTED_EDGE('',*,*,#11463,.F.);
#15919=ORIENTED_EDGE('',*,*,#11391,.F.);
#15920=ORIENTED_EDGE('',*,*,#11464,.F.);
#15921=ORIENTED_EDGE('',*,*,#11465,.F.);
#15922=ORIENTED_EDGE('',*,*,#11466,.F.);
#15923=ORIENTED_EDGE('',*,*,#11464,.T.);
#15924=ORIENTED_EDGE('',*,*,#11390,.F.);
#15925=ORIENTED_EDGE('',*,*,#11462,.F.);
#15926=ORIENTED_EDGE('',*,*,#11463,.T.);
#15927=ORIENTED_EDGE('',*,*,#11467,.F.);
#15928=ORIENTED_EDGE('',*,*,#11468,.T.);
#15929=ORIENTED_EDGE('',*,*,#11392,.F.);
#15930=ORIENTED_EDGE('',*,*,#11468,.F.);
#15931=ORIENTED_EDGE('',*,*,#11469,.F.);
#15932=ORIENTED_EDGE('',*,*,#11470,.T.);
#15933=ORIENTED_EDGE('',*,*,#11393,.F.);
#15934=ORIENTED_EDGE('',*,*,#11471,.F.);
#15935=ORIENTED_EDGE('',*,*,#11395,.F.);
#15936=ORIENTED_EDGE('',*,*,#11472,.F.);
#15937=ORIENTED_EDGE('',*,*,#11473,.F.);
#15938=ORIENTED_EDGE('',*,*,#11474,.F.);
#15939=ORIENTED_EDGE('',*,*,#11472,.T.);
#15940=ORIENTED_EDGE('',*,*,#11394,.F.);
#15941=ORIENTED_EDGE('',*,*,#11470,.F.);
#15942=ORIENTED_EDGE('',*,*,#11471,.T.);
#15943=ORIENTED_EDGE('',*,*,#11475,.F.);
#15944=ORIENTED_EDGE('',*,*,#11476,.T.);
#15945=ORIENTED_EDGE('',*,*,#11396,.F.);
#15946=ORIENTED_EDGE('',*,*,#11476,.F.);
#15947=ORIENTED_EDGE('',*,*,#11477,.F.);
#15948=ORIENTED_EDGE('',*,*,#11478,.T.);
#15949=ORIENTED_EDGE('',*,*,#11397,.F.);
#15950=ORIENTED_EDGE('',*,*,#11479,.F.);
#15951=ORIENTED_EDGE('',*,*,#11399,.F.);
#15952=ORIENTED_EDGE('',*,*,#11480,.F.);
#15953=ORIENTED_EDGE('',*,*,#11481,.F.);
#15954=ORIENTED_EDGE('',*,*,#11482,.F.);
#15955=ORIENTED_EDGE('',*,*,#11480,.T.);
#15956=ORIENTED_EDGE('',*,*,#11398,.F.);
#15957=ORIENTED_EDGE('',*,*,#11478,.F.);
#15958=ORIENTED_EDGE('',*,*,#11479,.T.);
#15959=ORIENTED_EDGE('',*,*,#11483,.F.);
#15960=ORIENTED_EDGE('',*,*,#11484,.T.);
#15961=ORIENTED_EDGE('',*,*,#11400,.F.);
#15962=ORIENTED_EDGE('',*,*,#11484,.F.);
#15963=ORIENTED_EDGE('',*,*,#11485,.F.);
#15964=ORIENTED_EDGE('',*,*,#11486,.T.);
#15965=ORIENTED_EDGE('',*,*,#11401,.F.);
#15966=ORIENTED_EDGE('',*,*,#11487,.F.);
#15967=ORIENTED_EDGE('',*,*,#11403,.F.);
#15968=ORIENTED_EDGE('',*,*,#11488,.F.);
#15969=ORIENTED_EDGE('',*,*,#11489,.F.);
#15970=ORIENTED_EDGE('',*,*,#11490,.F.);
#15971=ORIENTED_EDGE('',*,*,#11488,.T.);
#15972=ORIENTED_EDGE('',*,*,#11402,.F.);
#15973=ORIENTED_EDGE('',*,*,#11486,.F.);
#15974=ORIENTED_EDGE('',*,*,#11487,.T.);
#15975=ORIENTED_EDGE('',*,*,#11491,.F.);
#15976=ORIENTED_EDGE('',*,*,#11492,.T.);
#15977=ORIENTED_EDGE('',*,*,#11404,.F.);
#15978=ORIENTED_EDGE('',*,*,#11492,.F.);
#15979=ORIENTED_EDGE('',*,*,#11493,.F.);
#15980=ORIENTED_EDGE('',*,*,#11494,.T.);
#15981=ORIENTED_EDGE('',*,*,#11405,.F.);
#15982=ORIENTED_EDGE('',*,*,#11495,.F.);
#15983=ORIENTED_EDGE('',*,*,#11407,.F.);
#15984=ORIENTED_EDGE('',*,*,#11496,.F.);
#15985=ORIENTED_EDGE('',*,*,#11497,.F.);
#15986=ORIENTED_EDGE('',*,*,#11498,.F.);
#15987=ORIENTED_EDGE('',*,*,#11496,.T.);
#15988=ORIENTED_EDGE('',*,*,#11406,.F.);
#15989=ORIENTED_EDGE('',*,*,#11494,.F.);
#15990=ORIENTED_EDGE('',*,*,#11495,.T.);
#15991=ORIENTED_EDGE('',*,*,#11499,.F.);
#15992=ORIENTED_EDGE('',*,*,#11500,.T.);
#15993=ORIENTED_EDGE('',*,*,#11408,.F.);
#15994=ORIENTED_EDGE('',*,*,#11500,.F.);
#15995=ORIENTED_EDGE('',*,*,#11501,.F.);
#15996=ORIENTED_EDGE('',*,*,#11502,.T.);
#15997=ORIENTED_EDGE('',*,*,#11409,.F.);
#15998=ORIENTED_EDGE('',*,*,#11503,.F.);
#15999=ORIENTED_EDGE('',*,*,#11411,.F.);
#16000=ORIENTED_EDGE('',*,*,#11504,.F.);
#16001=ORIENTED_EDGE('',*,*,#11505,.F.);
#16002=ORIENTED_EDGE('',*,*,#11506,.F.);
#16003=ORIENTED_EDGE('',*,*,#11504,.T.);
#16004=ORIENTED_EDGE('',*,*,#11410,.F.);
#16005=ORIENTED_EDGE('',*,*,#11502,.F.);
#16006=ORIENTED_EDGE('',*,*,#11503,.T.);
#16007=ORIENTED_EDGE('',*,*,#11507,.F.);
#16008=ORIENTED_EDGE('',*,*,#11508,.T.);
#16009=ORIENTED_EDGE('',*,*,#11412,.F.);
#16010=ORIENTED_EDGE('',*,*,#11508,.F.);
#16011=ORIENTED_EDGE('',*,*,#11509,.F.);
#16012=ORIENTED_EDGE('',*,*,#11510,.T.);
#16013=ORIENTED_EDGE('',*,*,#11413,.F.);
#16014=ORIENTED_EDGE('',*,*,#11511,.F.);
#16015=ORIENTED_EDGE('',*,*,#11415,.F.);
#16016=ORIENTED_EDGE('',*,*,#11512,.F.);
#16017=ORIENTED_EDGE('',*,*,#11513,.F.);
#16018=ORIENTED_EDGE('',*,*,#11514,.F.);
#16019=ORIENTED_EDGE('',*,*,#11512,.T.);
#16020=ORIENTED_EDGE('',*,*,#11414,.F.);
#16021=ORIENTED_EDGE('',*,*,#11510,.F.);
#16022=ORIENTED_EDGE('',*,*,#11511,.T.);
#16023=ORIENTED_EDGE('',*,*,#11515,.F.);
#16024=ORIENTED_EDGE('',*,*,#11516,.T.);
#16025=ORIENTED_EDGE('',*,*,#11416,.F.);
#16026=ORIENTED_EDGE('',*,*,#11516,.F.);
#16027=ORIENTED_EDGE('',*,*,#11517,.F.);
#16028=ORIENTED_EDGE('',*,*,#11518,.T.);
#16029=ORIENTED_EDGE('',*,*,#11417,.F.);
#16030=ORIENTED_EDGE('',*,*,#11519,.F.);
#16031=ORIENTED_EDGE('',*,*,#11419,.F.);
#16032=ORIENTED_EDGE('',*,*,#11520,.F.);
#16033=ORIENTED_EDGE('',*,*,#11521,.F.);
#16034=ORIENTED_EDGE('',*,*,#11522,.F.);
#16035=ORIENTED_EDGE('',*,*,#11520,.T.);
#16036=ORIENTED_EDGE('',*,*,#11418,.F.);
#16037=ORIENTED_EDGE('',*,*,#11518,.F.);
#16038=ORIENTED_EDGE('',*,*,#11519,.T.);
#16039=ORIENTED_EDGE('',*,*,#11523,.F.);
#16040=ORIENTED_EDGE('',*,*,#11524,.T.);
#16041=ORIENTED_EDGE('',*,*,#11420,.F.);
#16042=ORIENTED_EDGE('',*,*,#11524,.F.);
#16043=ORIENTED_EDGE('',*,*,#11525,.F.);
#16044=ORIENTED_EDGE('',*,*,#11526,.T.);
#16045=ORIENTED_EDGE('',*,*,#11421,.F.);
#16046=ORIENTED_EDGE('',*,*,#11527,.F.);
#16047=ORIENTED_EDGE('',*,*,#11423,.F.);
#16048=ORIENTED_EDGE('',*,*,#11528,.F.);
#16049=ORIENTED_EDGE('',*,*,#11529,.F.);
#16050=ORIENTED_EDGE('',*,*,#11530,.F.);
#16051=ORIENTED_EDGE('',*,*,#11528,.T.);
#16052=ORIENTED_EDGE('',*,*,#11422,.F.);
#16053=ORIENTED_EDGE('',*,*,#11526,.F.);
#16054=ORIENTED_EDGE('',*,*,#11527,.T.);
#16055=ORIENTED_EDGE('',*,*,#11531,.F.);
#16056=ORIENTED_EDGE('',*,*,#11532,.T.);
#16057=ORIENTED_EDGE('',*,*,#11424,.F.);
#16058=ORIENTED_EDGE('',*,*,#11532,.F.);
#16059=ORIENTED_EDGE('',*,*,#11533,.F.);
#16060=ORIENTED_EDGE('',*,*,#11534,.T.);
#16061=ORIENTED_EDGE('',*,*,#11425,.F.);
#16062=ORIENTED_EDGE('',*,*,#11535,.F.);
#16063=ORIENTED_EDGE('',*,*,#11427,.F.);
#16064=ORIENTED_EDGE('',*,*,#11536,.F.);
#16065=ORIENTED_EDGE('',*,*,#11537,.F.);
#16066=ORIENTED_EDGE('',*,*,#11538,.F.);
#16067=ORIENTED_EDGE('',*,*,#11536,.T.);
#16068=ORIENTED_EDGE('',*,*,#11426,.F.);
#16069=ORIENTED_EDGE('',*,*,#11534,.F.);
#16070=ORIENTED_EDGE('',*,*,#11535,.T.);
#16071=ORIENTED_EDGE('',*,*,#11539,.F.);
#16072=ORIENTED_EDGE('',*,*,#11540,.T.);
#16073=ORIENTED_EDGE('',*,*,#11428,.F.);
#16074=ORIENTED_EDGE('',*,*,#11541,.F.);
#16075=ORIENTED_EDGE('',*,*,#11431,.F.);
#16076=ORIENTED_EDGE('',*,*,#11542,.F.);
#16077=ORIENTED_EDGE('',*,*,#11543,.F.);
#16078=ORIENTED_EDGE('',*,*,#11540,.F.);
#16079=ORIENTED_EDGE('',*,*,#11544,.F.);
#16080=ORIENTED_EDGE('',*,*,#11545,.T.);
#16081=ORIENTED_EDGE('',*,*,#11429,.F.);
#16082=ORIENTED_EDGE('',*,*,#11546,.F.);
#16083=ORIENTED_EDGE('',*,*,#11542,.T.);
#16084=ORIENTED_EDGE('',*,*,#11430,.F.);
#16085=ORIENTED_EDGE('',*,*,#11545,.F.);
#16086=ORIENTED_EDGE('',*,*,#11437,.T.);
#16087=ORIENTED_EDGE('',*,*,#11547,.T.);
#16088=ORIENTED_EDGE('',*,*,#11543,.T.);
#16089=ORIENTED_EDGE('',*,*,#11546,.T.);
#16090=ORIENTED_EDGE('',*,*,#11544,.T.);
#16091=ORIENTED_EDGE('',*,*,#11539,.T.);
#16092=ORIENTED_EDGE('',*,*,#11537,.T.);
#16093=ORIENTED_EDGE('',*,*,#11538,.T.);
#16094=ORIENTED_EDGE('',*,*,#11533,.T.);
#16095=ORIENTED_EDGE('',*,*,#11531,.T.);
#16096=ORIENTED_EDGE('',*,*,#11529,.T.);
#16097=ORIENTED_EDGE('',*,*,#11530,.T.);
#16098=ORIENTED_EDGE('',*,*,#11525,.T.);
#16099=ORIENTED_EDGE('',*,*,#11523,.T.);
#16100=ORIENTED_EDGE('',*,*,#11521,.T.);
#16101=ORIENTED_EDGE('',*,*,#11522,.T.);
#16102=ORIENTED_EDGE('',*,*,#11517,.T.);
#16103=ORIENTED_EDGE('',*,*,#11515,.T.);
#16104=ORIENTED_EDGE('',*,*,#11513,.T.);
#16105=ORIENTED_EDGE('',*,*,#11514,.T.);
#16106=ORIENTED_EDGE('',*,*,#11509,.T.);
#16107=ORIENTED_EDGE('',*,*,#11507,.T.);
#16108=ORIENTED_EDGE('',*,*,#11505,.T.);
#16109=ORIENTED_EDGE('',*,*,#11506,.T.);
#16110=ORIENTED_EDGE('',*,*,#11501,.T.);
#16111=ORIENTED_EDGE('',*,*,#11499,.T.);
#16112=ORIENTED_EDGE('',*,*,#11497,.T.);
#16113=ORIENTED_EDGE('',*,*,#11498,.T.);
#16114=ORIENTED_EDGE('',*,*,#11493,.T.);
#16115=ORIENTED_EDGE('',*,*,#11491,.T.);
#16116=ORIENTED_EDGE('',*,*,#11489,.T.);
#16117=ORIENTED_EDGE('',*,*,#11490,.T.);
#16118=ORIENTED_EDGE('',*,*,#11485,.T.);
#16119=ORIENTED_EDGE('',*,*,#11483,.T.);
#16120=ORIENTED_EDGE('',*,*,#11481,.T.);
#16121=ORIENTED_EDGE('',*,*,#11482,.T.);
#16122=ORIENTED_EDGE('',*,*,#11477,.T.);
#16123=ORIENTED_EDGE('',*,*,#11475,.T.);
#16124=ORIENTED_EDGE('',*,*,#11473,.T.);
#16125=ORIENTED_EDGE('',*,*,#11474,.T.);
#16126=ORIENTED_EDGE('',*,*,#11469,.T.);
#16127=ORIENTED_EDGE('',*,*,#11467,.T.);
#16128=ORIENTED_EDGE('',*,*,#11465,.T.);
#16129=ORIENTED_EDGE('',*,*,#11466,.T.);
#16130=ORIENTED_EDGE('',*,*,#11461,.T.);
#16131=ORIENTED_EDGE('',*,*,#11459,.T.);
#16132=ORIENTED_EDGE('',*,*,#11457,.T.);
#16133=ORIENTED_EDGE('',*,*,#11458,.T.);
#16134=ORIENTED_EDGE('',*,*,#11453,.T.);
#16135=ORIENTED_EDGE('',*,*,#11451,.T.);
#16136=ORIENTED_EDGE('',*,*,#11449,.T.);
#16137=ORIENTED_EDGE('',*,*,#11450,.T.);
#16138=ORIENTED_EDGE('',*,*,#11445,.T.);
#16139=ORIENTED_EDGE('',*,*,#11443,.T.);
#16140=ORIENTED_EDGE('',*,*,#11441,.T.);
#16141=ORIENTED_EDGE('',*,*,#11442,.T.);
#16142=ORIENTED_EDGE('',*,*,#11548,.F.);
#16143=ORIENTED_EDGE('',*,*,#11436,.T.);
#16144=ORIENTED_EDGE('',*,*,#11432,.F.);
#16145=ORIENTED_EDGE('',*,*,#11541,.T.);
#16146=ORIENTED_EDGE('',*,*,#11547,.F.);
#16147=ORIENTED_EDGE('',*,*,#11377,.F.);
#16148=ORIENTED_EDGE('',*,*,#11549,.T.);
#16149=ORIENTED_EDGE('',*,*,#11548,.T.);
#16150=ORIENTED_EDGE('',*,*,#11549,.F.);
#19554=ADVANCED_FACE('',(#5620),#230,.T.);
#19555=ADVANCED_FACE('',(#5621),#4801,.T.);
#19556=ADVANCED_FACE('',(#5622,#1754),#1477,.T.);
#19557=ADVANCED_FACE('',(#5623),#231,.T.);
#19558=ADVANCED_FACE('',(#5624,#1755),#1478,.T.);
#19559=ADVANCED_FACE('',(#5625),#1479,.T.);
#19560=ADVANCED_FACE('',(#5626),#1480,.T.);
#19561=ADVANCED_FACE('',(#5627),#1481,.T.);
#19562=ADVANCED_FACE('',(#5628),#4802,.F.);
#19563=ADVANCED_FACE('',(#5629),#1482,.T.);
#19564=ADVANCED_FACE('',(#5630),#1483,.T.);
#19565=ADVANCED_FACE('',(#5631),#1484,.T.);
#19566=ADVANCED_FACE('',(#5632),#4803,.F.);
#19567=ADVANCED_FACE('',(#5633),#1485,.T.);
#19568=ADVANCED_FACE('',(#5634),#1486,.T.);
#19569=ADVANCED_FACE('',(#5635),#1487,.T.);
#19570=ADVANCED_FACE('',(#5636),#4804,.F.);
#19571=ADVANCED_FACE('',(#5637),#1488,.T.);
#19572=ADVANCED_FACE('',(#5638),#1489,.T.);
#19573=ADVANCED_FACE('',(#5639),#1490,.T.);
#19574=ADVANCED_FACE('',(#5640),#4805,.F.);
#19575=ADVANCED_FACE('',(#5641),#1491,.T.);
#19576=ADVANCED_FACE('',(#5642),#1492,.T.);
#19577=ADVANCED_FACE('',(#5643),#1493,.T.);
#19578=ADVANCED_FACE('',(#5644),#4806,.F.);
#19579=ADVANCED_FACE('',(#5645),#1494,.T.);
#19580=ADVANCED_FACE('',(#5646),#1495,.T.);
#19581=ADVANCED_FACE('',(#5647),#1496,.T.);
#19582=ADVANCED_FACE('',(#5648),#4807,.F.);
#19583=ADVANCED_FACE('',(#5649),#1497,.T.);
#19584=ADVANCED_FACE('',(#5650),#1498,.T.);
#19585=ADVANCED_FACE('',(#5651),#1499,.T.);
#19586=ADVANCED_FACE('',(#5652),#4808,.F.);
#19587=ADVANCED_FACE('',(#5653),#1500,.T.);
#19588=ADVANCED_FACE('',(#5654),#1501,.T.);
#19589=ADVANCED_FACE('',(#5655),#1502,.T.);
#19590=ADVANCED_FACE('',(#5656),#4809,.F.);
#19591=ADVANCED_FACE('',(#5657),#1503,.T.);
#19592=ADVANCED_FACE('',(#5658),#1504,.T.);
#19593=ADVANCED_FACE('',(#5659),#1505,.T.);
#19594=ADVANCED_FACE('',(#5660),#4810,.F.);
#19595=ADVANCED_FACE('',(#5661),#1506,.T.);
#19596=ADVANCED_FACE('',(#5662),#1507,.T.);
#19597=ADVANCED_FACE('',(#5663),#1508,.T.);
#19598=ADVANCED_FACE('',(#5664),#4811,.F.);
#19599=ADVANCED_FACE('',(#5665),#1509,.T.);
#19600=ADVANCED_FACE('',(#5666),#1510,.T.);
#19601=ADVANCED_FACE('',(#5667),#1511,.T.);
#19602=ADVANCED_FACE('',(#5668),#4812,.F.);
#19603=ADVANCED_FACE('',(#5669),#1512,.T.);
#19604=ADVANCED_FACE('',(#5670),#1513,.T.);
#19605=ADVANCED_FACE('',(#5671),#1514,.T.);
#19606=ADVANCED_FACE('',(#5672),#4813,.F.);
#19607=ADVANCED_FACE('',(#5673),#1515,.T.);
#19608=ADVANCED_FACE('',(#5674),#1516,.T.);
#19609=ADVANCED_FACE('',(#5675),#1517,.T.);
#19610=ADVANCED_FACE('',(#5676),#4814,.F.);
#19611=ADVANCED_FACE('',(#5677),#1518,.T.);
#19612=ADVANCED_FACE('',(#5678),#1519,.T.);
#19613=ADVANCED_FACE('',(#5679),#1520,.T.);
#19614=ADVANCED_FACE('',(#5680,#1756),#1521,.T.);
#19615=ADVANCED_FACE('',(#5681),#4815,.F.);
#19616=ADVANCED_FACE('',(#5682),#4816,.F.);
#20121=CLOSED_SHELL('',(#19554,#19555,#19556,#19557,#19558,#19559,#19560,
#19561,#19562,#19563,#19564,#19565,#19566,#19567,#19568,#19569,#19570,#19571,
#19572,#19573,#19574,#19575,#19576,#19577,#19578,#19579,#19580,#19581,#19582,
#19583,#19584,#19585,#19586,#19587,#19588,#19589,#19590,#19591,#19592,#19593,
#19594,#19595,#19596,#19597,#19598,#19599,#19600,#19601,#19602,#19603,#19604,
#19605,#19606,#19607,#19608,#19609,#19610,#19611,#19612,#19613,#19614,#19615,
#19616));
#21437=AXIS2_PLACEMENT_3D('',#61626,#25347,#25348);
#21438=AXIS2_PLACEMENT_3D('',#61627,#25349,#25350);
#21439=AXIS2_PLACEMENT_3D('',#61630,#25351,#25352);
#21440=AXIS2_PLACEMENT_3D('',#61633,#25354,#25355);
#21441=AXIS2_PLACEMENT_3D('',#61634,#25356,#25357);
#21442=AXIS2_PLACEMENT_3D('',#61635,#25358,#25359);
#21443=AXIS2_PLACEMENT_3D('',#61638,#25360,#25361);
#21444=AXIS2_PLACEMENT_3D('',#61639,#25362,#25363);
#21445=AXIS2_PLACEMENT_3D('',#61641,#25365,#25366);
#21446=AXIS2_PLACEMENT_3D('',#61643,#25367,#25368);
#21447=AXIS2_PLACEMENT_3D('',#61644,#25369,#25370);
#21448=AXIS2_PLACEMENT_3D('',#61647,#25372,#25373);
#21449=AXIS2_PLACEMENT_3D('',#61648,#25374,#25375);
#21450=AXIS2_PLACEMENT_3D('',#61651,#25376,#25377);
#21451=AXIS2_PLACEMENT_3D('',#61659,#25381,#25382);
#21452=AXIS2_PLACEMENT_3D('',#61667,#25386,#25387);
#21453=AXIS2_PLACEMENT_3D('',#61675,#25391,#25392);
#21454=AXIS2_PLACEMENT_3D('',#61683,#25396,#25397);
#21455=AXIS2_PLACEMENT_3D('',#61691,#25401,#25402);
#21456=AXIS2_PLACEMENT_3D('',#61699,#25406,#25407);
#21457=AXIS2_PLACEMENT_3D('',#61707,#25411,#25412);
#21458=AXIS2_PLACEMENT_3D('',#61715,#25416,#25417);
#21459=AXIS2_PLACEMENT_3D('',#61723,#25421,#25422);
#21460=AXIS2_PLACEMENT_3D('',#61731,#25426,#25427);
#21461=AXIS2_PLACEMENT_3D('',#61739,#25431,#25432);
#21462=AXIS2_PLACEMENT_3D('',#61747,#25436,#25437);
#21463=AXIS2_PLACEMENT_3D('',#61755,#25441,#25442);
#21464=AXIS2_PLACEMENT_3D('',#61761,#25446,#25447);
#21465=AXIS2_PLACEMENT_3D('',#61767,#25451,#25452);
#21466=AXIS2_PLACEMENT_3D('',#61773,#25456,#25457);
#21467=AXIS2_PLACEMENT_3D('',#61775,#25459,#25460);
#21468=AXIS2_PLACEMENT_3D('',#61777,#25461,#25462);
#21469=AXIS2_PLACEMENT_3D('',#61779,#25464,#25465);
#21470=AXIS2_PLACEMENT_3D('',#61783,#25468,#25469);
#21471=AXIS2_PLACEMENT_3D('',#61789,#25473,#25474);
#21472=AXIS2_PLACEMENT_3D('',#61791,#25476,#25477);
#21473=AXIS2_PLACEMENT_3D('',#61793,#25478,#25479);
#21474=AXIS2_PLACEMENT_3D('',#61795,#25481,#25482);
#21475=AXIS2_PLACEMENT_3D('',#61799,#25485,#25486);
#21476=AXIS2_PLACEMENT_3D('',#61805,#25490,#25491);
#21477=AXIS2_PLACEMENT_3D('',#61807,#25493,#25494);
#21478=AXIS2_PLACEMENT_3D('',#61809,#25495,#25496);
#21479=AXIS2_PLACEMENT_3D('',#61811,#25498,#25499);
#21480=AXIS2_PLACEMENT_3D('',#61815,#25502,#25503);
#21481=AXIS2_PLACEMENT_3D('',#61821,#25507,#25508);
#21482=AXIS2_PLACEMENT_3D('',#61823,#25510,#25511);
#21483=AXIS2_PLACEMENT_3D('',#61825,#25512,#25513);
#21484=AXIS2_PLACEMENT_3D('',#61827,#25515,#25516);
#21485=AXIS2_PLACEMENT_3D('',#61831,#25519,#25520);
#21486=AXIS2_PLACEMENT_3D('',#61837,#25524,#25525);
#21487=AXIS2_PLACEMENT_3D('',#61839,#25527,#25528);
#21488=AXIS2_PLACEMENT_3D('',#61841,#25529,#25530);
#21489=AXIS2_PLACEMENT_3D('',#61843,#25532,#25533);
#21490=AXIS2_PLACEMENT_3D('',#61847,#25536,#25537);
#21491=AXIS2_PLACEMENT_3D('',#61853,#25541,#25542);
#21492=AXIS2_PLACEMENT_3D('',#61855,#25544,#25545);
#21493=AXIS2_PLACEMENT_3D('',#61857,#25546,#25547);
#21494=AXIS2_PLACEMENT_3D('',#61859,#25549,#25550);
#21495=AXIS2_PLACEMENT_3D('',#61863,#25553,#25554);
#21496=AXIS2_PLACEMENT_3D('',#61869,#25558,#25559);
#21497=AXIS2_PLACEMENT_3D('',#61871,#25561,#25562);
#21498=AXIS2_PLACEMENT_3D('',#61873,#25563,#25564);
#21499=AXIS2_PLACEMENT_3D('',#61875,#25566,#25567);
#21500=AXIS2_PLACEMENT_3D('',#61879,#25570,#25571);
#21501=AXIS2_PLACEMENT_3D('',#61885,#25575,#25576);
#21502=AXIS2_PLACEMENT_3D('',#61887,#25578,#25579);
#21503=AXIS2_PLACEMENT_3D('',#61889,#25580,#25581);
#21504=AXIS2_PLACEMENT_3D('',#61891,#25583,#25584);
#21505=AXIS2_PLACEMENT_3D('',#61895,#25587,#25588);
#21506=AXIS2_PLACEMENT_3D('',#61901,#25592,#25593);
#21507=AXIS2_PLACEMENT_3D('',#61903,#25595,#25596);
#21508=AXIS2_PLACEMENT_3D('',#61905,#25597,#25598);
#21509=AXIS2_PLACEMENT_3D('',#61907,#25600,#25601);
#21510=AXIS2_PLACEMENT_3D('',#61911,#25604,#25605);
#21511=AXIS2_PLACEMENT_3D('',#61917,#25609,#25610);
#21512=AXIS2_PLACEMENT_3D('',#61919,#25612,#25613);
#21513=AXIS2_PLACEMENT_3D('',#61921,#25614,#25615);
#21514=AXIS2_PLACEMENT_3D('',#61923,#25617,#25618);
#21515=AXIS2_PLACEMENT_3D('',#61927,#25621,#25622);
#21516=AXIS2_PLACEMENT_3D('',#61933,#25626,#25627);
#21517=AXIS2_PLACEMENT_3D('',#61935,#25629,#25630);
#21518=AXIS2_PLACEMENT_3D('',#61937,#25631,#25632);
#21519=AXIS2_PLACEMENT_3D('',#61939,#25634,#25635);
#21520=AXIS2_PLACEMENT_3D('',#61943,#25638,#25639);
#21521=AXIS2_PLACEMENT_3D('',#61949,#25643,#25644);
#21522=AXIS2_PLACEMENT_3D('',#61951,#25646,#25647);
#21523=AXIS2_PLACEMENT_3D('',#61953,#25648,#25649);
#21524=AXIS2_PLACEMENT_3D('',#61955,#25651,#25652);
#21525=AXIS2_PLACEMENT_3D('',#61959,#25655,#25656);
#21526=AXIS2_PLACEMENT_3D('',#61965,#25660,#25661);
#21527=AXIS2_PLACEMENT_3D('',#61967,#25663,#25664);
#21528=AXIS2_PLACEMENT_3D('',#61969,#25665,#25666);
#21529=AXIS2_PLACEMENT_3D('',#61971,#25668,#25669);
#21530=AXIS2_PLACEMENT_3D('',#61977,#25673,#25674);
#21531=AXIS2_PLACEMENT_3D('',#61981,#25677,#25678);
#21532=AXIS2_PLACEMENT_3D('',#61983,#25680,#25681);
#21533=AXIS2_PLACEMENT_3D('',#61984,#25682,#25683);
#21534=AXIS2_PLACEMENT_3D('',#61986,#25684,#25685);
#21535=AXIS2_PLACEMENT_3D('',#61987,#25686,#25687);
#21536=AXIS2_PLACEMENT_3D('',#61988,#25688,#25689);
#25347=DIRECTION('axis',(0.,0.,1.));
#25348=DIRECTION('refdir',(1.,0.,0.));
#25349=DIRECTION('center_axis',(1.,0.,0.));
#25350=DIRECTION('ref_axis',(0.,-1.,0.));
#25351=DIRECTION('center_axis',(-1.,0.,0.));
#25352=DIRECTION('ref_axis',(0.,-1.,0.));
#25353=DIRECTION('',(-0.707106781186548,-0.707106781186547,-8.65956056235493E-17));
#25354=DIRECTION('center_axis',(1.,0.,0.));
#25355=DIRECTION('ref_axis',(0.,-1.,0.));
#25356=DIRECTION('center_axis',(-1.,0.,0.));
#25357=DIRECTION('ref_axis',(0.,-1.,0.));
#25358=DIRECTION('center_axis',(1.,0.,0.));
#25359=DIRECTION('ref_axis',(0.,1.,0.));
#25360=DIRECTION('center_axis',(1.,0.,0.));
#25361=DIRECTION('ref_axis',(0.,-1.,0.));
#25362=DIRECTION('center_axis',(1.,0.,0.));
#25363=DIRECTION('ref_axis',(0.,-1.,0.));
#25364=DIRECTION('',(-1.,0.,0.));
#25365=DIRECTION('center_axis',(-1.,0.,0.));
#25366=DIRECTION('ref_axis',(0.,0.,1.));
#25367=DIRECTION('center_axis',(1.,0.,0.));
#25368=DIRECTION('ref_axis',(0.,0.,-1.));
#25369=DIRECTION('center_axis',(-1.,0.,0.));
#25370=DIRECTION('ref_axis',(0.,-1.,0.));
#25371=DIRECTION('',(0.707106781186548,-0.707106781186547,8.65956056235493E-17));
#25372=DIRECTION('center_axis',(-1.,0.,0.));
#25373=DIRECTION('ref_axis',(0.,-1.,0.));
#25374=DIRECTION('center_axis',(1.,0.,0.));
#25375=DIRECTION('ref_axis',(0.,0.,-1.));
#25376=DIRECTION('center_axis',(-1.,0.,0.));
#25377=DIRECTION('ref_axis',(0.,0.,-1.));
#25378=DIRECTION('',(0.,-0.668692731746348,-0.743538856085952));
#25379=DIRECTION('',(0.,0.623489801858733,-0.78183148246803));
#25380=DIRECTION('',(0.,0.873694915787935,0.486474248163572));
#25381=DIRECTION('center_axis',(-1.,0.,0.));
#25382=DIRECTION('ref_axis',(0.,0.,-1.));
#25383=DIRECTION('',(0.,-0.925080752553848,-0.37977045863838));
#25384=DIRECTION('',(0.,0.222520933956314,-0.974927912181824));
#25385=DIRECTION('',(0.,0.998245184947169,0.0592161357215442));
#25386=DIRECTION('center_axis',(-1.,0.,0.));
#25387=DIRECTION('ref_axis',(0.,0.,-1.));
#25388=DIRECTION('',(0.,-0.998245184947169,0.0592161357215445));
#25389=DIRECTION('',(0.,-0.222520933956315,-0.974927912181824));
#25390=DIRECTION('',(0.,0.925080752553848,-0.37977045863838));
#25391=DIRECTION('center_axis',(-1.,0.,0.));
#25392=DIRECTION('ref_axis',(0.,0.,-1.));
#25393=DIRECTION('',(0.,-0.873694915787935,0.486474248163572));
#25394=DIRECTION('',(0.,-0.623489801858734,-0.78183148246803));
#25395=DIRECTION('',(0.,0.668692731746348,-0.743538856085952));
#25396=DIRECTION('center_axis',(-1.,0.,0.));
#25397=DIRECTION('ref_axis',(0.,0.,-1.));
#25398=DIRECTION('',(0.,-0.576098653391942,0.817380169541683));
#25399=DIRECTION('',(0.,-0.900968867902419,-0.433883739117558));
#25400=DIRECTION('',(0.,0.279861914438318,-0.96004026418006));
#25401=DIRECTION('center_axis',(-1.,0.,0.));
#25402=DIRECTION('ref_axis',(0.,0.,-1.));
#25403=DIRECTION('',(0.,-0.164398987305357,0.986393923832144));
#25404=DIRECTION('',(0.,-1.,1.22464679914735E-16));
#25405=DIRECTION('',(0.,-0.164398987305357,-0.986393923832144));
#25406=DIRECTION('center_axis',(-1.,0.,0.));
#25407=DIRECTION('ref_axis',(0.,0.,-1.));
#25408=DIRECTION('',(0.,0.279861914438319,0.96004026418006));
#25409=DIRECTION('',(0.,-0.900968867902419,0.433883739117558));
#25410=DIRECTION('',(0.,-0.576098653391942,-0.817380169541683));
#25411=DIRECTION('center_axis',(-1.,0.,0.));
#25412=DIRECTION('ref_axis',(0.,0.,-1.));
#25413=DIRECTION('',(0.,0.668692731746348,0.743538856085952));
#25414=DIRECTION('',(0.,-0.623489801858733,0.78183148246803));
#25415=DIRECTION('',(0.,-0.873694915787935,-0.486474248163572));
#25416=DIRECTION('center_axis',(-1.,0.,0.));
#25417=DIRECTION('ref_axis',(0.,0.,-1.));
#25418=DIRECTION('',(0.,0.925080752553848,0.37977045863838));
#25419=DIRECTION('',(0.,-0.222520933956314,0.974927912181824));
#25420=DIRECTION('',(0.,-0.998245184947169,-0.0592161357215443));
#25421=DIRECTION('center_axis',(-1.,0.,0.));
#25422=DIRECTION('ref_axis',(0.,0.,-1.));
#25423=DIRECTION('',(0.,0.998245184947169,-0.0592161357215444));
#25424=DIRECTION('',(0.,0.222520933956314,0.974927912181824));
#25425=DIRECTION('',(0.,-0.925080752553848,0.37977045863838));
#25426=DIRECTION('center_axis',(-1.,0.,0.));
#25427=DIRECTION('ref_axis',(0.,0.,-1.));
#25428=DIRECTION('',(0.,0.873694915787935,-0.486474248163572));
#25429=DIRECTION('',(0.,0.623489801858734,0.78183148246803));
#25430=DIRECTION('',(0.,-0.668692731746348,0.743538856085952));
#25431=DIRECTION('center_axis',(-1.,0.,0.));
#25432=DIRECTION('ref_axis',(0.,0.,-1.));
#25433=DIRECTION('',(0.,0.576098653391942,-0.817380169541683));
#25434=DIRECTION('',(0.,0.900968867902419,0.433883739117558));
#25435=DIRECTION('',(0.,-0.279861914438319,0.96004026418006));
#25436=DIRECTION('center_axis',(-1.,0.,0.));
#25437=DIRECTION('ref_axis',(0.,0.,-1.));
#25438=DIRECTION('',(0.,0.164398987305357,-0.986393923832144));
#25439=DIRECTION('',(0.,1.,0.));
#25440=DIRECTION('',(0.,0.164398987305357,0.986393923832144));
#25441=DIRECTION('center_axis',(-1.,0.,0.));
#25442=DIRECTION('ref_axis',(0.,0.,-1.));
#25443=DIRECTION('',(0.,-0.279861914438319,-0.96004026418006));
#25444=DIRECTION('',(0.,0.900968867902419,-0.433883739117558));
#25445=DIRECTION('',(0.,0.576098653391942,0.817380169541683));
#25446=DIRECTION('center_axis',(0.,-0.96004026418006,0.279861914438319));
#25447=DIRECTION('ref_axis',(0.,-0.279861914438319,-0.96004026418006));
#25448=DIRECTION('',(1.,0.,0.));
#25449=DIRECTION('',(0.,0.279861914438319,0.96004026418006));
#25450=DIRECTION('',(1.,0.,0.));
#25451=DIRECTION('center_axis',(0.,0.817380169541683,-0.576098653391942));
#25452=DIRECTION('ref_axis',(0.,0.576098653391942,0.817380169541683));
#25453=DIRECTION('',(-1.,0.,0.));
#25454=DIRECTION('',(1.,0.,0.));
#25455=DIRECTION('',(0.,-0.576098653391942,-0.817380169541683));
#25456=DIRECTION('center_axis',(0.,-0.433883739117558,-0.900968867902419));
#25457=DIRECTION('ref_axis',(0.,0.900968867902419,-0.433883739117558));
#25458=DIRECTION('',(0.,-0.900968867902419,0.433883739117558));
#25459=DIRECTION('center_axis',(1.,0.,0.));
#25460=DIRECTION('ref_axis',(0.,0.,-1.));
#25461=DIRECTION('center_axis',(1.,0.,0.));
#25462=DIRECTION('ref_axis',(0.,0.,-1.));
#25463=DIRECTION('',(1.,0.,0.));
#25464=DIRECTION('center_axis',(0.,-0.743538856085952,0.668692731746348));
#25465=DIRECTION('ref_axis',(0.,-0.668692731746348,-0.743538856085952));
#25466=DIRECTION('',(0.,0.668692731746348,0.743538856085952));
#25467=DIRECTION('',(1.,0.,0.));
#25468=DIRECTION('center_axis',(0.,0.486474248163572,-0.873694915787935));
#25469=DIRECTION('ref_axis',(0.,0.873694915787935,0.486474248163572));
#25470=DIRECTION('',(-1.,0.,0.));
#25471=DIRECTION('',(1.,0.,0.));
#25472=DIRECTION('',(0.,-0.873694915787935,-0.486474248163572));
#25473=DIRECTION('center_axis',(0.,-0.78183148246803,-0.623489801858733));
#25474=DIRECTION('ref_axis',(0.,0.623489801858733,-0.78183148246803));
#25475=DIRECTION('',(0.,-0.623489801858733,0.78183148246803));
#25476=DIRECTION('center_axis',(1.,0.,0.));
#25477=DIRECTION('ref_axis',(0.,0.,-1.));
#25478=DIRECTION('center_axis',(1.,0.,0.));
#25479=DIRECTION('ref_axis',(0.,0.,-1.));
#25480=DIRECTION('',(1.,0.,0.));
#25481=DIRECTION('center_axis',(0.,-0.37977045863838,0.925080752553848));
#25482=DIRECTION('ref_axis',(0.,-0.925080752553848,-0.37977045863838));
#25483=DIRECTION('',(0.,0.925080752553848,0.37977045863838));
#25484=DIRECTION('',(1.,0.,0.));
#25485=DIRECTION('center_axis',(0.,0.0592161357215442,-0.998245184947169));
#25486=DIRECTION('ref_axis',(0.,0.998245184947169,0.0592161357215442));
#25487=DIRECTION('',(-1.,0.,0.));
#25488=DIRECTION('',(1.,0.,0.));
#25489=DIRECTION('',(0.,-0.998245184947169,-0.0592161357215442));
#25490=DIRECTION('center_axis',(0.,-0.974927912181824,-0.222520933956314));
#25491=DIRECTION('ref_axis',(0.,0.222520933956314,-0.974927912181824));
#25492=DIRECTION('',(0.,-0.222520933956314,0.974927912181824));
#25493=DIRECTION('center_axis',(1.,0.,0.));
#25494=DIRECTION('ref_axis',(0.,0.,-1.));
#25495=DIRECTION('center_axis',(1.,0.,0.));
#25496=DIRECTION('ref_axis',(0.,0.,-1.));
#25497=DIRECTION('',(1.,0.,0.));
#25498=DIRECTION('center_axis',(0.,0.0592161357215445,0.998245184947169));
#25499=DIRECTION('ref_axis',(0.,-0.998245184947169,0.0592161357215445));
#25500=DIRECTION('',(0.,0.998245184947169,-0.0592161357215445));
#25501=DIRECTION('',(1.,0.,0.));
#25502=DIRECTION('center_axis',(0.,-0.37977045863838,-0.925080752553848));
#25503=DIRECTION('ref_axis',(0.,0.925080752553848,-0.37977045863838));
#25504=DIRECTION('',(-1.,0.,0.));
#25505=DIRECTION('',(1.,0.,0.));
#25506=DIRECTION('',(0.,-0.925080752553848,0.37977045863838));
#25507=DIRECTION('center_axis',(0.,-0.974927912181824,0.222520933956315));
#25508=DIRECTION('ref_axis',(0.,-0.222520933956315,-0.974927912181824));
#25509=DIRECTION('',(0.,0.222520933956315,0.974927912181824));
#25510=DIRECTION('center_axis',(1.,0.,0.));
#25511=DIRECTION('ref_axis',(0.,0.,-1.));
#25512=DIRECTION('center_axis',(1.,0.,0.));
#25513=DIRECTION('ref_axis',(0.,0.,-1.));
#25514=DIRECTION('',(1.,0.,0.));
#25515=DIRECTION('center_axis',(0.,0.486474248163572,0.873694915787935));
#25516=DIRECTION('ref_axis',(0.,-0.873694915787935,0.486474248163572));
#25517=DIRECTION('',(0.,0.873694915787935,-0.486474248163572));
#25518=DIRECTION('',(1.,0.,0.));
#25519=DIRECTION('center_axis',(0.,-0.743538856085952,-0.668692731746348));
#25520=DIRECTION('ref_axis',(0.,0.668692731746348,-0.743538856085952));
#25521=DIRECTION('',(-1.,0.,0.));
#25522=DIRECTION('',(1.,0.,0.));
#25523=DIRECTION('',(0.,-0.668692731746348,0.743538856085952));
#25524=DIRECTION('center_axis',(0.,-0.78183148246803,0.623489801858734));
#25525=DIRECTION('ref_axis',(0.,-0.623489801858734,-0.78183148246803));
#25526=DIRECTION('',(0.,0.623489801858734,0.78183148246803));
#25527=DIRECTION('center_axis',(1.,0.,0.));
#25528=DIRECTION('ref_axis',(0.,0.,-1.));
#25529=DIRECTION('center_axis',(1.,0.,0.));
#25530=DIRECTION('ref_axis',(0.,0.,-1.));
#25531=DIRECTION('',(1.,0.,0.));
#25532=DIRECTION('center_axis',(0.,0.817380169541683,0.576098653391942));
#25533=DIRECTION('ref_axis',(0.,-0.576098653391942,0.817380169541683));
#25534=DIRECTION('',(0.,0.576098653391942,-0.817380169541683));
#25535=DIRECTION('',(1.,0.,0.));
#25536=DIRECTION('center_axis',(0.,-0.96004026418006,-0.279861914438318));
#25537=DIRECTION('ref_axis',(0.,0.279861914438318,-0.96004026418006));
#25538=DIRECTION('',(-1.,0.,0.));
#25539=DIRECTION('',(1.,0.,0.));
#25540=DIRECTION('',(0.,-0.279861914438318,0.96004026418006));
#25541=DIRECTION('center_axis',(0.,-0.433883739117558,0.900968867902419));
#25542=DIRECTION('ref_axis',(0.,-0.900968867902419,-0.433883739117558));
#25543=DIRECTION('',(0.,0.900968867902419,0.433883739117558));
#25544=DIRECTION('center_axis',(1.,0.,0.));
#25545=DIRECTION('ref_axis',(0.,0.,-1.));
#25546=DIRECTION('center_axis',(1.,0.,0.));
#25547=DIRECTION('ref_axis',(0.,0.,-1.));
#25548=DIRECTION('',(1.,0.,0.));
#25549=DIRECTION('center_axis',(0.,0.986393923832144,0.164398987305357));
#25550=DIRECTION('ref_axis',(0.,-0.164398987305357,0.986393923832144));
#25551=DIRECTION('',(0.,0.164398987305357,-0.986393923832144));
#25552=DIRECTION('',(1.,0.,0.));
#25553=DIRECTION('center_axis',(0.,-0.986393923832144,0.164398987305357));
#25554=DIRECTION('ref_axis',(0.,-0.164398987305357,-0.986393923832144));
#25555=DIRECTION('',(-1.,0.,0.));
#25556=DIRECTION('',(1.,0.,0.));
#25557=DIRECTION('',(0.,0.164398987305357,0.986393923832144));
#25558=DIRECTION('center_axis',(0.,1.22464679914735E-16,1.));
#25559=DIRECTION('ref_axis',(0.,-1.,1.22464679914735E-16));
#25560=DIRECTION('',(0.,1.,-1.22464679914735E-16));
#25561=DIRECTION('center_axis',(1.,0.,0.));
#25562=DIRECTION('ref_axis',(0.,0.,-1.));
#25563=DIRECTION('center_axis',(1.,0.,0.));
#25564=DIRECTION('ref_axis',(0.,0.,-1.));
#25565=DIRECTION('',(1.,0.,0.));
#25566=DIRECTION('center_axis',(0.,0.96004026418006,-0.279861914438319));
#25567=DIRECTION('ref_axis',(0.,0.279861914438319,0.96004026418006));
#25568=DIRECTION('',(0.,-0.279861914438319,-0.96004026418006));
#25569=DIRECTION('',(1.,0.,0.));
#25570=DIRECTION('center_axis',(0.,-0.817380169541683,0.576098653391942));
#25571=DIRECTION('ref_axis',(0.,-0.576098653391942,-0.817380169541683));
#25572=DIRECTION('',(-1.,0.,0.));
#25573=DIRECTION('',(1.,0.,0.));
#25574=DIRECTION('',(0.,0.576098653391942,0.817380169541683));
#25575=DIRECTION('center_axis',(0.,0.433883739117558,0.900968867902419));
#25576=DIRECTION('ref_axis',(0.,-0.900968867902419,0.433883739117558));
#25577=DIRECTION('',(0.,0.900968867902419,-0.433883739117558));
#25578=DIRECTION('center_axis',(1.,0.,0.));
#25579=DIRECTION('ref_axis',(0.,0.,-1.));
#25580=DIRECTION('center_axis',(1.,0.,0.));
#25581=DIRECTION('ref_axis',(0.,0.,-1.));
#25582=DIRECTION('',(1.,0.,0.));
#25583=DIRECTION('center_axis',(0.,0.743538856085952,-0.668692731746348));
#25584=DIRECTION('ref_axis',(0.,0.668692731746348,0.743538856085952));
#25585=DIRECTION('',(0.,-0.668692731746348,-0.743538856085952));
#25586=DIRECTION('',(1.,0.,0.));
#25587=DIRECTION('center_axis',(0.,-0.486474248163572,0.873694915787935));
#25588=DIRECTION('ref_axis',(0.,-0.873694915787935,-0.486474248163572));
#25589=DIRECTION('',(-1.,0.,0.));
#25590=DIRECTION('',(1.,0.,0.));
#25591=DIRECTION('',(0.,0.873694915787935,0.486474248163572));
#25592=DIRECTION('center_axis',(0.,0.78183148246803,0.623489801858733));
#25593=DIRECTION('ref_axis',(0.,-0.623489801858733,0.78183148246803));
#25594=DIRECTION('',(0.,0.623489801858733,-0.78183148246803));
#25595=DIRECTION('center_axis',(1.,0.,0.));
#25596=DIRECTION('ref_axis',(0.,0.,-1.));
#25597=DIRECTION('center_axis',(1.,0.,0.));
#25598=DIRECTION('ref_axis',(0.,0.,-1.));
#25599=DIRECTION('',(1.,0.,0.));
#25600=DIRECTION('center_axis',(0.,0.37977045863838,-0.925080752553848));
#25601=DIRECTION('ref_axis',(0.,0.925080752553848,0.37977045863838));
#25602=DIRECTION('',(0.,-0.925080752553848,-0.37977045863838));
#25603=DIRECTION('',(1.,0.,0.));
#25604=DIRECTION('center_axis',(0.,-0.0592161357215443,0.998245184947169));
#25605=DIRECTION('ref_axis',(0.,-0.998245184947169,-0.0592161357215443));
#25606=DIRECTION('',(-1.,0.,0.));
#25607=DIRECTION('',(1.,0.,0.));
#25608=DIRECTION('',(0.,0.998245184947169,0.0592161357215443));
#25609=DIRECTION('center_axis',(0.,0.974927912181824,0.222520933956314));
#25610=DIRECTION('ref_axis',(0.,-0.222520933956314,0.974927912181824));
#25611=DIRECTION('',(0.,0.222520933956314,-0.974927912181824));
#25612=DIRECTION('center_axis',(1.,0.,0.));
#25613=DIRECTION('ref_axis',(0.,0.,-1.));
#25614=DIRECTION('center_axis',(1.,0.,0.));
#25615=DIRECTION('ref_axis',(0.,0.,-1.));
#25616=DIRECTION('',(1.,0.,0.));
#25617=DIRECTION('center_axis',(0.,-0.0592161357215444,-0.998245184947169));
#25618=DIRECTION('ref_axis',(0.,0.998245184947169,-0.0592161357215444));
#25619=DIRECTION('',(0.,-0.998245184947169,0.0592161357215444));
#25620=DIRECTION('',(1.,0.,0.));
#25621=DIRECTION('center_axis',(0.,0.37977045863838,0.925080752553848));
#25622=DIRECTION('ref_axis',(0.,-0.925080752553848,0.37977045863838));
#25623=DIRECTION('',(-1.,0.,0.));
#25624=DIRECTION('',(1.,0.,0.));
#25625=DIRECTION('',(0.,0.925080752553848,-0.37977045863838));
#25626=DIRECTION('center_axis',(0.,0.974927912181824,-0.222520933956314));
#25627=DIRECTION('ref_axis',(0.,0.222520933956314,0.974927912181824));
#25628=DIRECTION('',(0.,-0.222520933956314,-0.974927912181824));
#25629=DIRECTION('center_axis',(1.,0.,0.));
#25630=DIRECTION('ref_axis',(0.,0.,-1.));
#25631=DIRECTION('center_axis',(1.,0.,0.));
#25632=DIRECTION('ref_axis',(0.,0.,-1.));
#25633=DIRECTION('',(1.,0.,0.));
#25634=DIRECTION('center_axis',(0.,-0.486474248163572,-0.873694915787935));
#25635=DIRECTION('ref_axis',(0.,0.873694915787935,-0.486474248163572));
#25636=DIRECTION('',(0.,-0.873694915787935,0.486474248163572));
#25637=DIRECTION('',(1.,0.,0.));
#25638=DIRECTION('center_axis',(0.,0.743538856085952,0.668692731746348));
#25639=DIRECTION('ref_axis',(0.,-0.668692731746348,0.743538856085952));
#25640=DIRECTION('',(-1.,0.,0.));
#25641=DIRECTION('',(1.,0.,0.));
#25642=DIRECTION('',(0.,0.668692731746348,-0.743538856085952));
#25643=DIRECTION('center_axis',(0.,0.78183148246803,-0.623489801858734));
#25644=DIRECTION('ref_axis',(0.,0.623489801858734,0.78183148246803));
#25645=DIRECTION('',(0.,-0.623489801858734,-0.78183148246803));
#25646=DIRECTION('center_axis',(1.,0.,0.));
#25647=DIRECTION('ref_axis',(0.,0.,-1.));
#25648=DIRECTION('center_axis',(1.,0.,0.));
#25649=DIRECTION('ref_axis',(0.,0.,-1.));
#25650=DIRECTION('',(1.,0.,0.));
#25651=DIRECTION('center_axis',(0.,-0.817380169541683,-0.576098653391942));
#25652=DIRECTION('ref_axis',(0.,0.576098653391942,-0.817380169541683));
#25653=DIRECTION('',(0.,-0.576098653391942,0.817380169541683));
#25654=DIRECTION('',(1.,0.,0.));
#25655=DIRECTION('center_axis',(0.,0.96004026418006,0.279861914438319));
#25656=DIRECTION('ref_axis',(0.,-0.279861914438319,0.96004026418006));
#25657=DIRECTION('',(-1.,0.,0.));
#25658=DIRECTION('',(1.,0.,0.));
#25659=DIRECTION('',(0.,0.279861914438319,-0.96004026418006));
#25660=DIRECTION('center_axis',(0.,0.433883739117558,-0.900968867902419));
#25661=DIRECTION('ref_axis',(0.,0.900968867902419,0.433883739117558));
#25662=DIRECTION('',(0.,-0.900968867902419,-0.433883739117558));
#25663=DIRECTION('center_axis',(1.,0.,0.));
#25664=DIRECTION('ref_axis',(0.,0.,-1.));
#25665=DIRECTION('center_axis',(1.,0.,0.));
#25666=DIRECTION('ref_axis',(0.,0.,-1.));
#25667=DIRECTION('',(1.,0.,0.));
#25668=DIRECTION('center_axis',(0.,0.986393923832144,-0.164398987305357));
#25669=DIRECTION('ref_axis',(0.,0.164398987305357,0.986393923832144));
#25670=DIRECTION('',(-1.,0.,0.));
#25671=DIRECTION('',(1.,0.,0.));
#25672=DIRECTION('',(0.,-0.164398987305357,-0.986393923832144));
#25673=DIRECTION('center_axis',(0.,-0.986393923832144,-0.164398987305357));
#25674=DIRECTION('ref_axis',(0.,0.164398987305357,-0.986393923832144));
#25675=DIRECTION('',(0.,-0.164398987305357,0.986393923832144));
#25676=DIRECTION('',(1.,0.,0.));
#25677=DIRECTION('center_axis',(0.,0.,-1.));
#25678=DIRECTION('ref_axis',(0.,1.,0.));
#25679=DIRECTION('',(0.,-1.,0.));
#25680=DIRECTION('center_axis',(1.,0.,0.));
#25681=DIRECTION('ref_axis',(0.,0.,-1.));
#25682=DIRECTION('center_axis',(1.,0.,0.));
#25683=DIRECTION('ref_axis',(0.,0.,-1.));
#25684=DIRECTION('center_axis',(1.,0.,0.));
#25685=DIRECTION('ref_axis',(0.,1.,0.));
#25686=DIRECTION('center_axis',(1.,0.,0.));
#25687=DIRECTION('ref_axis',(0.,0.,-1.));
#25688=DIRECTION('center_axis',(1.,0.,0.));
#25689=DIRECTION('ref_axis',(0.,1.,0.));
#25690=DIRECTION('',(1.,0.,0.));
#61626=CARTESIAN_POINT('',(0.,0.,0.));
#61627=CARTESIAN_POINT('Origin',(0.1632,0.,0.));
#61628=CARTESIAN_POINT('',(0.326400000000001,-5.712,-6.99518251672968E-16));
#61629=CARTESIAN_POINT('',(0.3264,5.712,6.99518251672968E-16));
#61630=CARTESIAN_POINT('Origin',(0.3264,0.,0.));
#61631=CARTESIAN_POINT('',(0.,5.3856,6.59545780148798E-16));
#61632=CARTESIAN_POINT('',(0.1632,5.5488,6.79532015910883E-16));
#61633=CARTESIAN_POINT('Origin',(0.,0.,0.));
#61634=CARTESIAN_POINT('Origin',(0.3264,0.,0.));
#61635=CARTESIAN_POINT('Origin',(3.264,0.,0.));
#61636=CARTESIAN_POINT('',(6.0384,5.712,6.99518251672968E-16));
#61637=CARTESIAN_POINT('',(6.0384,-5.712,-6.99518251672968E-16));
#61638=CARTESIAN_POINT('Origin',(6.0384,0.,0.));
#61639=CARTESIAN_POINT('Origin',(6.0384,0.,0.));
#61640=CARTESIAN_POINT('',(3.264,-5.712,-6.99518251672968E-16));
#61641=CARTESIAN_POINT('Origin',(0.,5.712,0.));
#61642=CARTESIAN_POINT('',(0.,-2.448,-2.99793536431272E-16));
#61643=CARTESIAN_POINT('Origin',(0.,0.,0.));
#61644=CARTESIAN_POINT('Origin',(6.2832,0.,0.));
#61645=CARTESIAN_POINT('',(6.528,5.2224,-6.39559544386714E-16));
#61646=CARTESIAN_POINT('',(6.2832,5.4672,-6.69538898029841E-16));
#61647=CARTESIAN_POINT('Origin',(6.528,0.,0.));
#61648=CARTESIAN_POINT('Origin',(6.528,2.448,0.));
#61649=CARTESIAN_POINT('',(6.528,2.51932419206087,3.71418222699114));
#61650=CARTESIAN_POINT('',(6.528,3.06045755186719,3.28264277270907));
#61651=CARTESIAN_POINT('Origin',(6.528,0.,0.));
#61652=CARTESIAN_POINT('',(6.528,2.54018621271673,2.70413797072631));
#61653=CARTESIAN_POINT('',(6.528,3.20400206468608,3.44225408264517));
#61654=CARTESIAN_POINT('',(6.528,3.20158419452848,1.87477113412423));
#61655=CARTESIAN_POINT('',(6.528,2.54018621271673,2.70413797072631));
#61656=CARTESIAN_POINT('',(6.528,3.88135593761115,2.2532687557348));
#61657=CARTESIAN_POINT('',(6.528,3.20158419452848,1.87477113412423));
#61658=CARTESIAN_POINT('',(6.528,4.18166229617943,1.62967617664105));
#61659=CARTESIAN_POINT('Origin',(6.528,0.,0.));
#61660=CARTESIAN_POINT('',(6.528,3.46191019016123,1.33419863410882));
#61661=CARTESIAN_POINT('',(6.528,4.380244185348,1.71119936790692));
#61662=CARTESIAN_POINT('',(6.528,3.69796039690208,0.299995104866347));
#61663=CARTESIAN_POINT('',(6.528,3.46191019016123,1.33419863410882));
#61664=CARTESIAN_POINT('',(6.528,4.47463753801084,0.346067772877413));
#61665=CARTESIAN_POINT('',(6.528,3.69796039690208,0.299995104866347));
#61666=CARTESIAN_POINT('',(6.528,4.47463753801084,-0.346067772877415));
#61667=CARTESIAN_POINT('Origin',(6.528,0.,0.));
#61668=CARTESIAN_POINT('',(6.528,3.69796039690209,-0.299995104866348));
#61669=CARTESIAN_POINT('',(6.528,4.6889252249322,-0.358779368128298));
#61670=CARTESIAN_POINT('',(6.528,3.46191019016123,-1.33419863410883));
#61671=CARTESIAN_POINT('',(6.528,3.69796039690209,-0.299995104866348));
#61672=CARTESIAN_POINT('',(6.528,4.18166229617943,-1.62967617664105));
#61673=CARTESIAN_POINT('',(6.528,3.46191019016123,-1.33419863410883));
#61674=CARTESIAN_POINT('',(6.528,3.88135593761115,-2.2532687557348));
#61675=CARTESIAN_POINT('Origin',(6.528,0.,0.));
#61676=CARTESIAN_POINT('',(6.528,3.20158419452848,-1.87477113412423));
#61677=CARTESIAN_POINT('',(6.528,4.06890711782452,-2.35769745016552));
#61678=CARTESIAN_POINT('',(6.528,2.54018621271673,-2.70413797072631));
#61679=CARTESIAN_POINT('',(6.528,3.20158419452848,-1.87477113412423));
#61680=CARTESIAN_POINT('',(6.528,3.06045755186718,-3.28264277270907));
#61681=CARTESIAN_POINT('',(6.528,2.54018621271673,-2.70413797072631));
#61682=CARTESIAN_POINT('',(6.528,2.51932419206087,-3.71418222699114));
#61683=CARTESIAN_POINT('Origin',(6.528,0.,0.));
#61684=CARTESIAN_POINT('',(6.528,2.07109497757512,-3.07822574770973));
#61685=CARTESIAN_POINT('',(6.528,2.6429920541607,-3.88964463693579));
#61686=CARTESIAN_POINT('',(6.528,1.11534720250423,-3.53848961816564));
#61687=CARTESIAN_POINT('',(6.528,2.07109497757512,-3.07822574770973));
#61688=CARTESIAN_POINT('',(6.528,1.33309165535894,-4.28544170867046));
#61689=CARTESIAN_POINT('',(6.528,1.11534720250423,-3.53848961816564));
#61690=CARTESIAN_POINT('',(6.528,0.658309392789363,-4.43945635673618));
#61691=CARTESIAN_POINT('Origin',(6.528,0.,0.));
#61692=CARTESIAN_POINT('',(6.528,0.5304,-3.672));
#61693=CARTESIAN_POINT('',(6.528,0.693599999999999,-4.6512));
#61694=CARTESIAN_POINT('',(6.528,-0.5304,-3.672));
#61695=CARTESIAN_POINT('',(6.528,0.5304,-3.672));
#61696=CARTESIAN_POINT('',(6.528,-0.658309392789364,-4.43945635673618));
#61697=CARTESIAN_POINT('',(6.528,-0.5304,-3.672));
#61698=CARTESIAN_POINT('',(6.528,-1.33309165535895,-4.28544170867045));
#61699=CARTESIAN_POINT('Origin',(6.528,0.,0.));
#61700=CARTESIAN_POINT('',(6.528,-1.11534720250423,-3.53848961816564));
#61701=CARTESIAN_POINT('',(6.528,-1.39316804060647,-4.49152815983967));
#61702=CARTESIAN_POINT('',(6.528,-2.07109497757512,-3.07822574770973));
#61703=CARTESIAN_POINT('',(6.528,-1.11534720250423,-3.53848961816564));
#61704=CARTESIAN_POINT('',(6.528,-2.51932419206087,-3.71418222699114));
#61705=CARTESIAN_POINT('',(6.528,-2.07109497757512,-3.07822574770973));
#61706=CARTESIAN_POINT('',(6.528,-3.06045755186719,-3.28264277270907));
#61707=CARTESIAN_POINT('Origin',(6.528,0.,0.));
#61708=CARTESIAN_POINT('',(6.528,-2.54018621271673,-2.70413797072631));
#61709=CARTESIAN_POINT('',(6.528,-3.20400206468608,-3.44225408264517));
#61710=CARTESIAN_POINT('',(6.528,-3.20158419452848,-1.87477113412423));
#61711=CARTESIAN_POINT('',(6.528,-2.54018621271673,-2.70413797072631));
#61712=CARTESIAN_POINT('',(6.528,-3.88135593761115,-2.2532687557348));
#61713=CARTESIAN_POINT('',(6.528,-3.20158419452848,-1.87477113412423));
#61714=CARTESIAN_POINT('',(6.528,-4.18166229617943,-1.62967617664105));
#61715=CARTESIAN_POINT('Origin',(6.528,0.,0.));
#61716=CARTESIAN_POINT('',(6.528,-3.46191019016123,-1.33419863410883));
#61717=CARTESIAN_POINT('',(6.528,-4.380244185348,-1.71119936790692));
#61718=CARTESIAN_POINT('',(6.528,-3.69796039690208,-0.299995104866347));
#61719=CARTESIAN_POINT('',(6.528,-3.46191019016123,-1.33419863410883));
#61720=CARTESIAN_POINT('',(6.528,-4.47463753801084,-0.346067772877414));
#61721=CARTESIAN_POINT('',(6.528,-3.69796039690209,-0.299995104866347));
#61722=CARTESIAN_POINT('',(6.528,-4.47463753801084,0.346067772877414));
#61723=CARTESIAN_POINT('Origin',(6.528,0.,0.));
#61724=CARTESIAN_POINT('',(6.528,-3.69796039690209,0.299995104866347));
#61725=CARTESIAN_POINT('',(6.528,-4.6889252249322,0.358779368128297));
#61726=CARTESIAN_POINT('',(6.528,-3.46191019016123,1.33419863410883));
#61727=CARTESIAN_POINT('',(6.528,-3.69796039690209,0.299995104866347));
#61728=CARTESIAN_POINT('',(6.528,-4.18166229617943,1.62967617664105));
#61729=CARTESIAN_POINT('',(6.528,-3.46191019016123,1.33419863410883));
#61730=CARTESIAN_POINT('',(6.528,-3.88135593761115,2.2532687557348));
#61731=CARTESIAN_POINT('Origin',(6.528,0.,0.));
#61732=CARTESIAN_POINT('',(6.528,-3.20158419452848,1.87477113412423));
#61733=CARTESIAN_POINT('',(6.528,-4.06890711782452,2.35769745016552));
#61734=CARTESIAN_POINT('',(6.528,-2.54018621271673,2.70413797072631));
#61735=CARTESIAN_POINT('',(6.528,-3.20158419452848,1.87477113412423));
#61736=CARTESIAN_POINT('',(6.528,-3.06045755186718,3.28264277270907));
#61737=CARTESIAN_POINT('',(6.528,-2.54018621271673,2.70413797072631));
#61738=CARTESIAN_POINT('',(6.528,-2.51932419206087,3.71418222699114));
#61739=CARTESIAN_POINT('Origin',(6.528,0.,0.));
#61740=CARTESIAN_POINT('',(6.528,-2.07109497757512,3.07822574770973));
#61741=CARTESIAN_POINT('',(6.528,-2.6429920541607,3.88964463693579));
#61742=CARTESIAN_POINT('',(6.528,-1.11534720250423,3.53848961816564));
#61743=CARTESIAN_POINT('',(6.528,-2.07109497757512,3.07822574770973));
#61744=CARTESIAN_POINT('',(6.528,-1.33309165535894,4.28544170867046));
#61745=CARTESIAN_POINT('',(6.528,-1.11534720250423,3.53848961816564));
#61746=CARTESIAN_POINT('',(6.528,-0.658309392789364,4.43945635673618));
#61747=CARTESIAN_POINT('Origin',(6.528,0.,0.));
#61748=CARTESIAN_POINT('',(6.528,-0.5304,3.672));
#61749=CARTESIAN_POINT('',(6.528,-0.6936,4.6512));
#61750=CARTESIAN_POINT('',(6.528,0.5304,3.672));
#61751=CARTESIAN_POINT('',(6.528,-0.5304,3.672));
#61752=CARTESIAN_POINT('',(6.528,0.658309392789364,4.43945635673618));
#61753=CARTESIAN_POINT('',(6.528,0.5304,3.672));
#61754=CARTESIAN_POINT('',(6.528,1.33309165535895,4.28544170867045));
#61755=CARTESIAN_POINT('Origin',(6.528,0.,0.));
#61756=CARTESIAN_POINT('',(6.528,1.11534720250423,3.53848961816564));
#61757=CARTESIAN_POINT('',(6.528,1.39316804060647,4.49152815983967));
#61758=CARTESIAN_POINT('',(6.528,2.07109497757512,3.07822574770973));
#61759=CARTESIAN_POINT('',(6.528,1.11534720250423,3.53848961816564));
#61760=CARTESIAN_POINT('',(6.528,2.07109497757512,3.07822574770973));
#61761=CARTESIAN_POINT('Origin',(1.632,1.39316804060647,4.49152815983967));
#61762=CARTESIAN_POINT('',(1.632,1.33309165535895,4.28544170867045));
#61763=CARTESIAN_POINT('',(1.632,1.33309165535895,4.28544170867045));
#61764=CARTESIAN_POINT('',(1.632,1.11534720250423,3.53848961816564));
#61765=CARTESIAN_POINT('',(1.632,0.735220717938668,2.23450107296974));
#61766=CARTESIAN_POINT('',(1.632,1.11534720250423,3.53848961816564));
#61767=CARTESIAN_POINT('Origin',(1.632,2.07109497757512,3.07822574770973));
#61768=CARTESIAN_POINT('',(1.632,2.51932419206087,3.71418222699114));
#61769=CARTESIAN_POINT('',(1.632,2.51932419206087,3.71418222699114));
#61770=CARTESIAN_POINT('',(1.632,2.07109497757512,3.07822574770973));
#61771=CARTESIAN_POINT('',(1.632,2.07109497757512,3.07822574770973));
#61772=CARTESIAN_POINT('',(1.632,1.00265212841353,1.5622978904732));
#61773=CARTESIAN_POINT('Origin',(1.632,1.11534720250423,3.53848961816564));
#61774=CARTESIAN_POINT('',(1.632,1.35428414627195,3.42342365055166));
#61775=CARTESIAN_POINT('Origin',(1.632,0.,0.));
#61776=CARTESIAN_POINT('',(1.632,3.06045755186719,3.28264277270907));
#61777=CARTESIAN_POINT('Origin',(1.632,0.,0.));
#61778=CARTESIAN_POINT('',(1.632,3.06045755186719,3.28264277270907));
#61779=CARTESIAN_POINT('Origin',(1.632,3.20400206468608,3.44225408264517));
#61780=CARTESIAN_POINT('',(1.632,2.54018621271673,2.70413797072631));
#61781=CARTESIAN_POINT('',(1.632,1.63192465850191,1.69421558786437));
#61782=CARTESIAN_POINT('',(1.632,2.54018621271673,2.70413797072631));
#61783=CARTESIAN_POINT('Origin',(1.632,3.20158419452848,1.87477113412423));
#61784=CARTESIAN_POINT('',(1.632,3.88135593761115,2.2532687557348));
#61785=CARTESIAN_POINT('',(1.632,3.88135593761115,2.2532687557348));
#61786=CARTESIAN_POINT('',(1.632,3.20158419452848,1.87477113412423));
#61787=CARTESIAN_POINT('',(1.632,3.20158419452848,1.87477113412423));
#61788=CARTESIAN_POINT('',(1.632,1.58121400337067,0.972547307195736));
#61789=CARTESIAN_POINT('Origin',(1.632,2.54018621271673,2.70413797072631));
#61790=CARTESIAN_POINT('',(1.632,2.70553570816967,2.49679626157579));
#61791=CARTESIAN_POINT('Origin',(1.632,0.,0.));
#61792=CARTESIAN_POINT('',(1.632,4.18166229617943,1.62967617664105));
#61793=CARTESIAN_POINT('Origin',(1.632,0.,0.));
#61794=CARTESIAN_POINT('',(1.632,4.18166229617943,1.62967617664105));
#61795=CARTESIAN_POINT('Origin',(1.632,4.380244185348,1.71119936790692));
#61796=CARTESIAN_POINT('',(1.632,3.46191019016123,1.33419863410882));
#61797=CARTESIAN_POINT('',(1.632,2.20540590620635,0.818369927391835));
#61798=CARTESIAN_POINT('',(1.632,3.46191019016123,1.33419863410882));
#61799=CARTESIAN_POINT('Origin',(1.632,3.69796039690208,0.299995104866347));
#61800=CARTESIAN_POINT('',(1.632,4.47463753801084,0.346067772877413));
#61801=CARTESIAN_POINT('',(1.632,4.47463753801084,0.346067772877413));
#61802=CARTESIAN_POINT('',(1.632,3.69796039690208,0.299995104866347));
#61803=CARTESIAN_POINT('',(1.632,3.69796039690208,0.299995104866347));
#61804=CARTESIAN_POINT('',(1.632,1.84659705264313,0.190171802218178));
#61805=CARTESIAN_POINT('Origin',(1.632,3.46191019016123,1.33419863410882));
#61806=CARTESIAN_POINT('',(1.632,3.52092274184644,1.07564775179821));
#61807=CARTESIAN_POINT('Origin',(1.632,0.,0.));
#61808=CARTESIAN_POINT('',(1.632,4.47463753801084,-0.346067772877415));
#61809=CARTESIAN_POINT('Origin',(1.632,0.,0.));
#61810=CARTESIAN_POINT('',(1.632,4.47463753801084,-0.346067772877415));
#61811=CARTESIAN_POINT('Origin',(1.632,4.6889252249322,-0.358779368128298));
#61812=CARTESIAN_POINT('',(1.632,3.69796039690209,-0.299995104866348));
#61813=CARTESIAN_POINT('',(1.632,2.34207946665818,-0.219563933849153));
#61814=CARTESIAN_POINT('',(1.632,3.69796039690209,-0.299995104866348));
#61815=CARTESIAN_POINT('Origin',(1.632,3.46191019016123,-1.33419863410883));
#61816=CARTESIAN_POINT('',(1.632,4.18166229617943,-1.62967617664105));
#61817=CARTESIAN_POINT('',(1.632,4.18166229617943,-1.62967617664105));
#61818=CARTESIAN_POINT('',(1.632,3.46191019016123,-1.33419863410883));
#61819=CARTESIAN_POINT('',(1.632,3.46191019016123,-1.33419863410883));
#61820=CARTESIAN_POINT('',(1.632,1.74623890861297,-0.629869560492788));
#61821=CARTESIAN_POINT('Origin',(1.632,3.69796039690209,-0.299995104866348));
#61822=CARTESIAN_POINT('',(1.632,3.63894784521687,-0.558545987176968));
#61823=CARTESIAN_POINT('Origin',(1.632,0.,0.));
#61824=CARTESIAN_POINT('',(1.632,3.88135593761115,-2.2532687557348));
#61825=CARTESIAN_POINT('Origin',(1.632,0.,0.));
#61826=CARTESIAN_POINT('',(1.632,3.88135593761115,-2.2532687557348));
#61827=CARTESIAN_POINT('Origin',(1.632,4.06890711782452,-2.35769745016552));
#61828=CARTESIAN_POINT('',(1.632,3.20158419452848,-1.87477113412423));
#61829=CARTESIAN_POINT('',(1.632,2.01487546501869,-1.21401046521638));
#61830=CARTESIAN_POINT('',(1.632,3.20158419452848,-1.87477113412423));
#61831=CARTESIAN_POINT('Origin',(1.632,2.54018621271673,-2.70413797072631));
#61832=CARTESIAN_POINT('',(1.632,3.06045755186718,-3.28264277270907));
#61833=CARTESIAN_POINT('',(1.632,3.06045755186718,-3.28264277270907));
#61834=CARTESIAN_POINT('',(1.632,2.54018621271673,-2.70413797072631));
#61835=CARTESIAN_POINT('',(1.632,2.54018621271673,-2.70413797072631));
#61836=CARTESIAN_POINT('',(1.632,1.30001673251724,-1.32515753190494));
#61837=CARTESIAN_POINT('Origin',(1.632,3.20158419452848,-1.87477113412423));
#61838=CARTESIAN_POINT('',(1.632,3.03623469907554,-2.08211284327475));
#61839=CARTESIAN_POINT('Origin',(1.632,0.,0.));
#61840=CARTESIAN_POINT('',(1.632,2.51932419206087,-3.71418222699114));
#61841=CARTESIAN_POINT('Origin',(1.632,0.,0.));
#61842=CARTESIAN_POINT('',(1.632,2.51932419206087,-3.71418222699114));
#61843=CARTESIAN_POINT('Origin',(1.632,2.6429920541607,-3.88964463693579));
#61844=CARTESIAN_POINT('',(1.632,2.07109497757512,-3.07822574770973));
#61845=CARTESIAN_POINT('',(1.632,1.28860066670632,-1.96800733508623));
#61846=CARTESIAN_POINT('',(1.632,2.07109497757512,-3.07822574770973));
#61847=CARTESIAN_POINT('Origin',(1.632,1.11534720250423,-3.53848961816564));
#61848=CARTESIAN_POINT('',(1.632,1.33309165535894,-4.28544170867046));
#61849=CARTESIAN_POINT('',(1.632,1.33309165535894,-4.28544170867046));
#61850=CARTESIAN_POINT('',(1.632,1.11534720250423,-3.53848961816564));
#61851=CARTESIAN_POINT('',(1.632,1.11534720250423,-3.53848961816564));
#61852=CARTESIAN_POINT('',(1.632,0.596310298887548,-1.75798180213273));
#61853=CARTESIAN_POINT('Origin',(1.632,2.07109497757512,-3.07822574770973));
#61854=CARTESIAN_POINT('',(1.632,1.83215803380739,-3.19329171532371));
#61855=CARTESIAN_POINT('Origin',(1.632,0.,0.));
#61856=CARTESIAN_POINT('',(1.632,0.658309392789363,-4.43945635673618));
#61857=CARTESIAN_POINT('Origin',(1.632,0.,0.));
#61858=CARTESIAN_POINT('',(1.632,0.658309392789363,-4.43945635673618));
#61859=CARTESIAN_POINT('Origin',(1.632,0.693599999999999,-4.6512));
#61860=CARTESIAN_POINT('',(1.632,0.5304,-3.672));
#61861=CARTESIAN_POINT('',(1.632,0.307102702702703,-2.33221621621622));
#61862=CARTESIAN_POINT('',(1.632,0.5304,-3.672));
#61863=CARTESIAN_POINT('Origin',(1.632,-0.5304,-3.672));
#61864=CARTESIAN_POINT('',(1.632,-0.658309392789364,-4.43945635673618));
#61865=CARTESIAN_POINT('',(1.632,-0.658309392789364,-4.43945635673618));
#61866=CARTESIAN_POINT('',(1.632,-0.5304,-3.672));
#61867=CARTESIAN_POINT('',(1.632,-0.5304,-3.672));
#61868=CARTESIAN_POINT('',(1.632,-0.225502702702703,-1.84261621621622));
#61869=CARTESIAN_POINT('Origin',(1.632,0.5304,-3.672));
#61870=CARTESIAN_POINT('',(1.632,0.2652,-3.672));
#61871=CARTESIAN_POINT('Origin',(1.632,0.,0.));
#61872=CARTESIAN_POINT('',(1.632,-1.33309165535895,-4.28544170867045));
#61873=CARTESIAN_POINT('Origin',(1.632,0.,0.));
#61874=CARTESIAN_POINT('',(1.632,-1.33309165535895,-4.28544170867045));
#61875=CARTESIAN_POINT('Origin',(1.632,-1.39316804060647,-4.49152815983967));
#61876=CARTESIAN_POINT('',(1.632,-1.11534720250423,-3.53848961816564));
#61877=CARTESIAN_POINT('',(1.632,-0.735220717938668,-2.23450107296974));
#61878=CARTESIAN_POINT('',(1.632,-1.11534720250423,-3.53848961816564));
#61879=CARTESIAN_POINT('Origin',(1.632,-2.07109497757512,-3.07822574770973));
#61880=CARTESIAN_POINT('',(1.632,-2.51932419206087,-3.71418222699114));
#61881=CARTESIAN_POINT('',(1.632,-2.51932419206087,-3.71418222699114));
#61882=CARTESIAN_POINT('',(1.632,-2.07109497757512,-3.07822574770973));
#61883=CARTESIAN_POINT('',(1.632,-2.07109497757512,-3.07822574770973));
#61884=CARTESIAN_POINT('',(1.632,-1.00265212841353,-1.5622978904732));
#61885=CARTESIAN_POINT('Origin',(1.632,-1.11534720250423,-3.53848961816564));
#61886=CARTESIAN_POINT('',(1.632,-1.35428414627195,-3.42342365055166));
#61887=CARTESIAN_POINT('Origin',(1.632,0.,0.));
#61888=CARTESIAN_POINT('',(1.632,-3.06045755186719,-3.28264277270907));
#61889=CARTESIAN_POINT('Origin',(1.632,0.,0.));
#61890=CARTESIAN_POINT('',(1.632,-3.06045755186719,-3.28264277270907));
#61891=CARTESIAN_POINT('Origin',(1.632,-3.20400206468608,-3.44225408264517));
#61892=CARTESIAN_POINT('',(1.632,-2.54018621271673,-2.70413797072631));
#61893=CARTESIAN_POINT('',(1.632,-1.63192465850191,-1.69421558786437));
#61894=CARTESIAN_POINT('',(1.632,-2.54018621271673,-2.70413797072631));
#61895=CARTESIAN_POINT('Origin',(1.632,-3.20158419452848,-1.87477113412423));
#61896=CARTESIAN_POINT('',(1.632,-3.88135593761115,-2.2532687557348));
#61897=CARTESIAN_POINT('',(1.632,-3.88135593761115,-2.2532687557348));
#61898=CARTESIAN_POINT('',(1.632,-3.20158419452848,-1.87477113412423));
#61899=CARTESIAN_POINT('',(1.632,-3.20158419452848,-1.87477113412423));
#61900=CARTESIAN_POINT('',(1.632,-1.58121400337067,-0.972547307195736));
#61901=CARTESIAN_POINT('Origin',(1.632,-2.54018621271673,-2.70413797072631));
#61902=CARTESIAN_POINT('',(1.632,-2.70553570816967,-2.49679626157579));
#61903=CARTESIAN_POINT('Origin',(1.632,0.,0.));
#61904=CARTESIAN_POINT('',(1.632,-4.18166229617943,-1.62967617664105));
#61905=CARTESIAN_POINT('Origin',(1.632,0.,0.));
#61906=CARTESIAN_POINT('',(1.632,-4.18166229617943,-1.62967617664105));
#61907=CARTESIAN_POINT('Origin',(1.632,-4.380244185348,-1.71119936790692));
#61908=CARTESIAN_POINT('',(1.632,-3.46191019016123,-1.33419863410883));
#61909=CARTESIAN_POINT('',(1.632,-2.20540590620635,-0.818369927391835));
#61910=CARTESIAN_POINT('',(1.632,-3.46191019016123,-1.33419863410883));
#61911=CARTESIAN_POINT('Origin',(1.632,-3.69796039690209,-0.299995104866347));
#61912=CARTESIAN_POINT('',(1.632,-4.47463753801084,-0.346067772877414));
#61913=CARTESIAN_POINT('',(1.632,-4.47463753801084,-0.346067772877414));
#61914=CARTESIAN_POINT('',(1.632,-3.69796039690209,-0.299995104866347));
#61915=CARTESIAN_POINT('',(1.632,-3.69796039690209,-0.299995104866347));
#61916=CARTESIAN_POINT('',(1.632,-1.84659705264313,-0.190171802218178));
#61917=CARTESIAN_POINT('Origin',(1.632,-3.46191019016123,-1.33419863410883));
#61918=CARTESIAN_POINT('',(1.632,-3.52092274184644,-1.07564775179821));
#61919=CARTESIAN_POINT('Origin',(1.632,0.,0.));
#61920=CARTESIAN_POINT('',(1.632,-4.47463753801084,0.346067772877414));
#61921=CARTESIAN_POINT('Origin',(1.632,0.,0.));
#61922=CARTESIAN_POINT('',(1.632,-4.47463753801084,0.346067772877414));
#61923=CARTESIAN_POINT('Origin',(1.632,-4.6889252249322,0.358779368128297));
#61924=CARTESIAN_POINT('',(1.632,-3.69796039690209,0.299995104866347));
#61925=CARTESIAN_POINT('',(1.632,-2.34207946665818,0.219563933849153));
#61926=CARTESIAN_POINT('',(1.632,-3.69796039690209,0.299995104866347));
#61927=CARTESIAN_POINT('Origin',(1.632,-3.46191019016123,1.33419863410883));
#61928=CARTESIAN_POINT('',(1.632,-4.18166229617943,1.62967617664105));
#61929=CARTESIAN_POINT('',(1.632,-4.18166229617943,1.62967617664105));
#61930=CARTESIAN_POINT('',(1.632,-3.46191019016123,1.33419863410883));
#61931=CARTESIAN_POINT('',(1.632,-3.46191019016123,1.33419863410883));
#61932=CARTESIAN_POINT('',(1.632,-1.74623890861297,0.629869560492787));
#61933=CARTESIAN_POINT('Origin',(1.632,-3.69796039690209,0.299995104866347));
#61934=CARTESIAN_POINT('',(1.632,-3.63894784521687,0.558545987176967));
#61935=CARTESIAN_POINT('Origin',(1.632,0.,0.));
#61936=CARTESIAN_POINT('',(1.632,-3.88135593761115,2.2532687557348));
#61937=CARTESIAN_POINT('Origin',(1.632,0.,0.));
#61938=CARTESIAN_POINT('',(1.632,-3.88135593761115,2.2532687557348));
#61939=CARTESIAN_POINT('Origin',(1.632,-4.06890711782452,2.35769745016552));
#61940=CARTESIAN_POINT('',(1.632,-3.20158419452848,1.87477113412423));
#61941=CARTESIAN_POINT('',(1.632,-2.01487546501869,1.21401046521638));
#61942=CARTESIAN_POINT('',(1.632,-3.20158419452848,1.87477113412423));
#61943=CARTESIAN_POINT('Origin',(1.632,-2.54018621271673,2.70413797072631));
#61944=CARTESIAN_POINT('',(1.632,-3.06045755186718,3.28264277270907));
#61945=CARTESIAN_POINT('',(1.632,-3.06045755186718,3.28264277270907));
#61946=CARTESIAN_POINT('',(1.632,-2.54018621271673,2.70413797072631));
#61947=CARTESIAN_POINT('',(1.632,-2.54018621271673,2.70413797072631));
#61948=CARTESIAN_POINT('',(1.632,-1.30001673251724,1.32515753190494));
#61949=CARTESIAN_POINT('Origin',(1.632,-3.20158419452848,1.87477113412423));
#61950=CARTESIAN_POINT('',(1.632,-3.03623469907554,2.08211284327475));
#61951=CARTESIAN_POINT('Origin',(1.632,0.,0.));
#61952=CARTESIAN_POINT('',(1.632,-2.51932419206087,3.71418222699114));
#61953=CARTESIAN_POINT('Origin',(1.632,0.,0.));
#61954=CARTESIAN_POINT('',(1.632,-2.51932419206087,3.71418222699114));
#61955=CARTESIAN_POINT('Origin',(1.632,-2.6429920541607,3.88964463693579));
#61956=CARTESIAN_POINT('',(1.632,-2.07109497757512,3.07822574770973));
#61957=CARTESIAN_POINT('',(1.632,-1.28860066670632,1.96800733508623));
#61958=CARTESIAN_POINT('',(1.632,-2.07109497757512,3.07822574770973));
#61959=CARTESIAN_POINT('Origin',(1.632,-1.11534720250423,3.53848961816564));
#61960=CARTESIAN_POINT('',(1.632,-1.33309165535894,4.28544170867046));
#61961=CARTESIAN_POINT('',(1.632,-1.33309165535894,4.28544170867046));
#61962=CARTESIAN_POINT('',(1.632,-1.11534720250423,3.53848961816564));
#61963=CARTESIAN_POINT('',(1.632,-1.11534720250423,3.53848961816564));
#61964=CARTESIAN_POINT('',(1.632,-0.596310298887548,1.75798180213273));
#61965=CARTESIAN_POINT('Origin',(1.632,-2.07109497757512,3.07822574770973));
#61966=CARTESIAN_POINT('',(1.632,-1.83215803380739,3.19329171532371));
#61967=CARTESIAN_POINT('Origin',(1.632,0.,0.));
#61968=CARTESIAN_POINT('',(1.632,-0.658309392789364,4.43945635673618));
#61969=CARTESIAN_POINT('Origin',(1.632,0.,0.));
#61970=CARTESIAN_POINT('',(1.632,-0.658309392789364,4.43945635673618));
#61971=CARTESIAN_POINT('Origin',(1.632,0.5304,3.672));
#61972=CARTESIAN_POINT('',(1.632,0.658309392789364,4.43945635673618));
#61973=CARTESIAN_POINT('',(1.632,0.658309392789364,4.43945635673618));
#61974=CARTESIAN_POINT('',(1.632,0.5304,3.672));
#61975=CARTESIAN_POINT('',(1.632,0.5304,3.672));
#61976=CARTESIAN_POINT('',(1.632,0.225502702702703,1.84261621621622));
#61977=CARTESIAN_POINT('Origin',(1.632,-0.6936,4.6512));
#61978=CARTESIAN_POINT('',(1.632,-0.5304,3.672));
#61979=CARTESIAN_POINT('',(1.632,-0.307102702702703,2.33221621621622));
#61980=CARTESIAN_POINT('',(1.632,-0.5304,3.672));
#61981=CARTESIAN_POINT('Origin',(1.632,-0.5304,3.672));
#61982=CARTESIAN_POINT('',(1.632,-0.2652,3.672));
#61983=CARTESIAN_POINT('Origin',(1.632,0.,0.));
#61984=CARTESIAN_POINT('Origin',(1.632,0.,0.));
#61985=CARTESIAN_POINT('',(1.632,-2.448,-2.99793536431272E-16));
#61986=CARTESIAN_POINT('Origin',(1.632,0.,0.));
#61987=CARTESIAN_POINT('Origin',(1.632,0.,0.));
#61988=CARTESIAN_POINT('Origin',(3.264,0.,0.));
#61989=CARTESIAN_POINT('',(3.264,-2.448,-2.99793536431272E-16));
#99997=UNCERTAINTY_MEASURE_WITH_UNIT(LENGTH_MEASURE(0.01),#100032,
'DISTANCE_ACCURACY_VALUE',
'Maximum model space distance between geometric entities at asserted c
onnectivities');
#100011=UNCERTAINTY_MEASURE_WITH_UNIT(LENGTH_MEASURE(0.01),#100032,
'DISTANCE_ACCURACY_VALUE',
'Maximum model space distance between geometric entities at asserted c
onnectivities');
#100017=(
GEOMETRIC_REPRESENTATION_CONTEXT(3)
GLOBAL_UNCERTAINTY_ASSIGNED_CONTEXT((#99997))
GLOBAL_UNIT_ASSIGNED_CONTEXT((#100032,#100034,#100035))
REPRESENTATION_CONTEXT('','3D')
);
#100031=(
GEOMETRIC_REPRESENTATION_CONTEXT(3)
GLOBAL_UNCERTAINTY_ASSIGNED_CONTEXT((#100011))
GLOBAL_UNIT_ASSIGNED_CONTEXT((#100032,#100034,#100035))
REPRESENTATION_CONTEXT('','3D')
);
#100032=(
LENGTH_UNIT()
NAMED_UNIT(*)
SI_UNIT(.MILLI.,.METRE.)
);
#100034=(
NAMED_UNIT(*)
PLANE_ANGLE_UNIT()
SI_UNIT($,.RADIAN.)
);
#100035=(
NAMED_UNIT(*)
SI_UNIT($,.STERADIAN.)
SOLID_ANGLE_UNIT()
);
#100041=SHAPE_DEFINITION_REPRESENTATION(#100060,#100105);
#100060=PRODUCT_DEFINITION_SHAPE('',$,#100125);
#100105=SHAPE_REPRESENTATION('',(#21437),#100017);
#100119=PRODUCT_DEFINITION_CONTEXT('part definition',#100178,'design');
#100125=PRODUCT_DEFINITION('2026-10-12-11-54-59-762',
'05_Input_Spline_Bush_14T',#100144,#100119);
#100144=PRODUCT_DEFINITION_FORMATION('',$,#100185);
#100178=APPLICATION_CONTEXT(
'Core Data for Automotive Mechanical Design Process');
#100179=PRODUCT_CONTEXT('part definition',#100178,'mechanical');
#100185=PRODUCT('2026-10-12-11-54-59-762','05_Input_Spline_Bush_14T',$,
(#100179));
#100200=PRESENTATION_STYLE_ASSIGNMENT((#100206));
#100206=SURFACE_STYLE_USAGE(.BOTH.,#100212);
#100212=SURFACE_SIDE_STYLE('',(#100218));
#100218=SURFACE_STYLE_FILL_AREA(#100224);
#100224=FILL_AREA_STYLE('Opaque(227,224,212)',(#100230));
#100230=FILL_AREA_STYLE_COLOUR('Opaque(227,224,212)',#100236);
#100236=COLOUR_RGB('Opaque(227,224,212)',0.890196078431372,0.87843137254902,
0.831372549019608);
ENDSEC;
END-ISO-10303-21;
